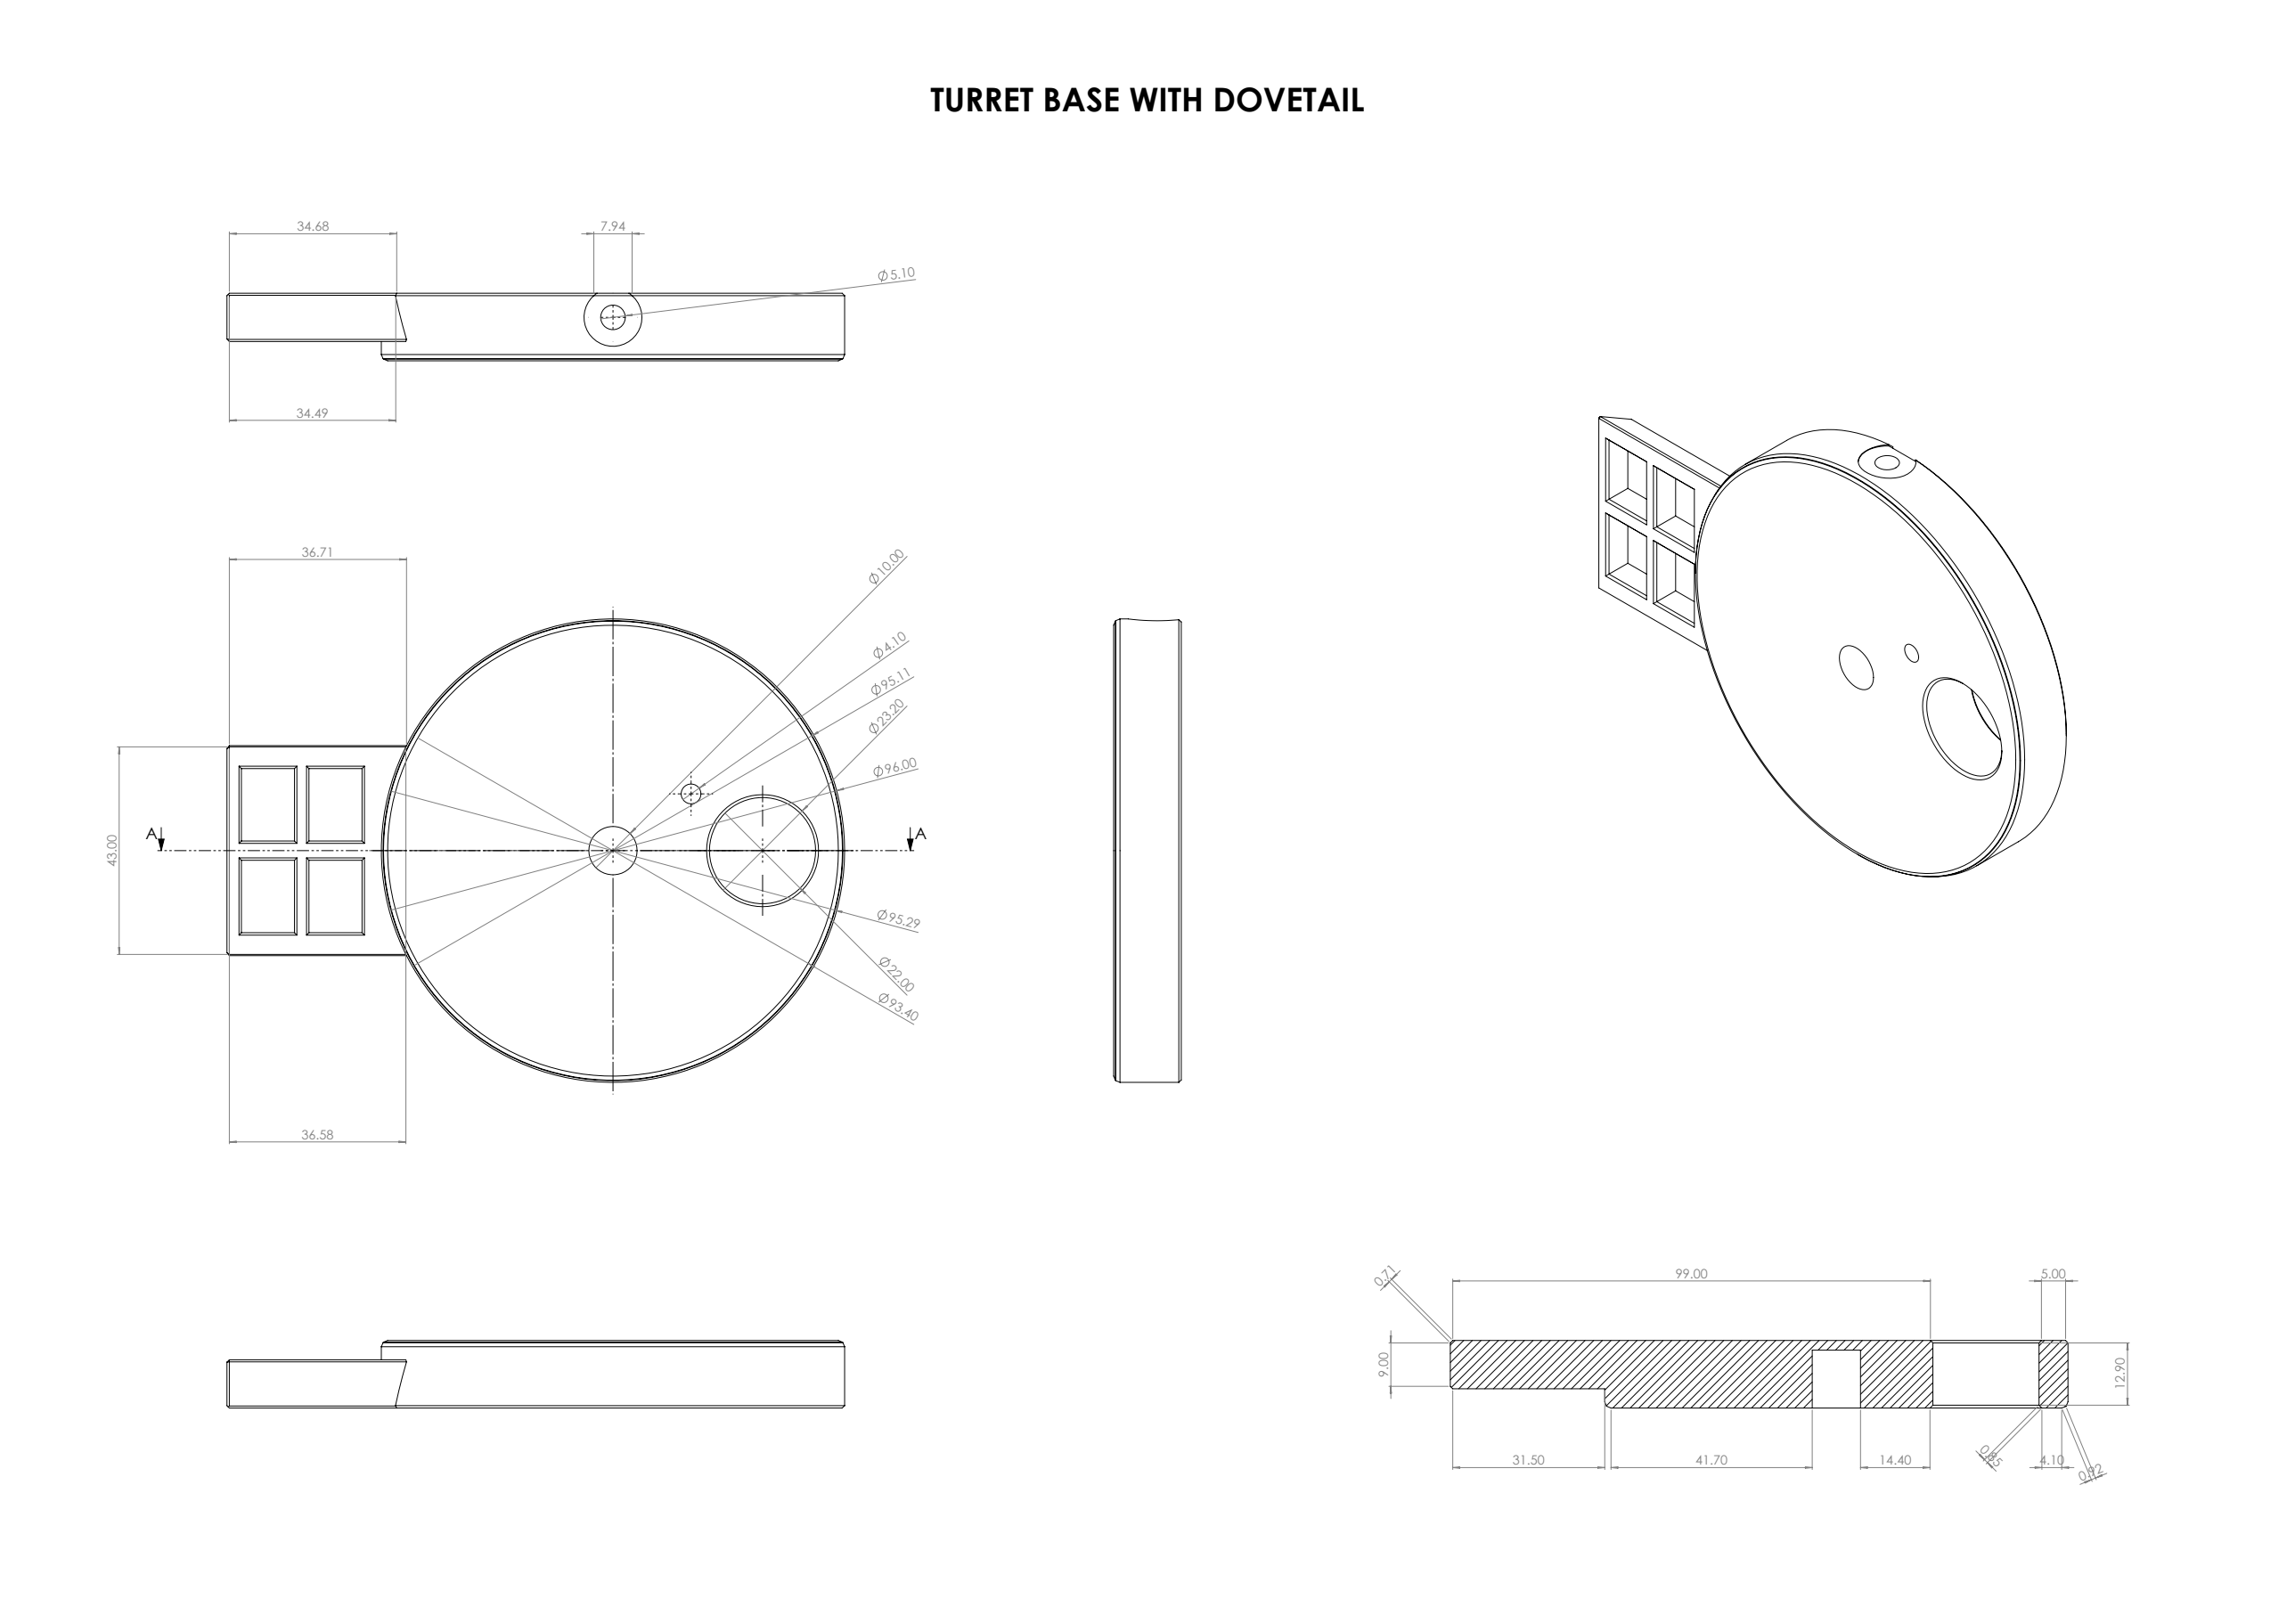
ISO-10303-21;
HEADER;
/* Generated by software containing ST-Developer
 * from STEP Tools, Inc. (www.steptools.com) 
 */

FILE_DESCRIPTION(
/* description */ (''),
/* implementation_level */ '2;1');

FILE_NAME(
/* name */ '01_Turret_Base_with_Dovetail.step',
/* time_stamp */ '2026-10-21T02:03:06-07:00',
/* author */ (''),
/* organization */ (''),
/* preprocessor_version */ 'ST-DEVELOPER v20.2',
/* originating_system */ 'Autodesk Translation Framework v15.15.0.0',
/* authorisation */ '');

FILE_SCHEMA (('AUTOMOTIVE_DESIGN { 1 0 10303 214 3 1 1 }'));
ENDSEC;

DATA;
#10=MECHANICAL_DESIGN_GEOMETRIC_PRESENTATION_REPRESENTATION('',(#115),#38528);
#91=SHAPE_REPRESENTATION_RELATIONSHIP('SRR','None',#38576,#103);
#103=ADVANCED_BREP_SHAPE_REPRESENTATION('',(#127),#38516);
#115=STYLED_ITEM('',(#38685),#127);
#127=MANIFOLD_SOLID_BREP('Body1',#17072);
#139=CYLINDRICAL_SURFACE('',#17258,6.);
#140=CYLINDRICAL_SURFACE('',#17281,2.55);
#141=CYLINDRICAL_SURFACE('',#17296,48.);
#142=CYLINDRICAL_SURFACE('',#17299,11.);
#143=CYLINDRICAL_SURFACE('',#17308,2.55);
#144=CYLINDRICAL_SURFACE('',#17313,2.05);
#145=CYLINDRICAL_SURFACE('',#17314,5.);
#428=B_SPLINE_CURVE_WITH_KNOTS('',3,(#23818,#23819,#23820,#23821,#23822,
#23823),.UNSPECIFIED.,.F.,.F.,(4,2,4),(2.30648016522772,2.36442361206073,
2.39897284114794),.UNSPECIFIED.);
#429=B_SPLINE_CURVE_WITH_KNOTS('',3,(#23838,#23839,#23840,#23841,#23842,
#23843),.UNSPECIFIED.,.F.,.F.,(4,2,4),(1.51323695998699,1.54778618907421,
1.60572963590723),.UNSPECIFIED.);
#430=B_SPLINE_CURVE_WITH_KNOTS('',3,(#23844,#23845,#23846,#23847,#23848,
#23849,#23850,#23851,#23852,#23853,#23854,#23855,#23856,#23857,#23858,#23859,
#23860,#23861,#23862,#23863,#23864,#23865,#23866,#23867,#23868,#23869,#23870,
#23871,#23872,#23873,#23874),.UNSPECIFIED.,.F.,.F.,(4,2,2,3,2,2,2,2,2,2,
2,2,2,2,4),(-0.489813721019733,-0.452534469426352,-0.226267234713176,0.,
0.226267234713176,0.452534469426352,0.678799813883625,0.905065158340898,
1.13133050279817,1.35759584725544,1.58386308196862,1.8101303166818,2.03639755139497,
2.26266478610815,2.29994403770815),.UNSPECIFIED.);
#847=CONICAL_SURFACE('',#17255,47.75,0.785398163397447);
#848=CONICAL_SURFACE('',#17266,47.75,0.785398163397447);
#849=CONICAL_SURFACE('',#17279,2.8,0.785398163397449);
#850=CONICAL_SURFACE('',#17291,47.8232233047034,0.392699081698724);
#851=CONICAL_SURFACE('',#17294,47.6,0.785398163397448);
#852=CONICAL_SURFACE('',#17297,11.25,0.785398163397446);
#853=CONICAL_SURFACE('',#17301,47.1267766952966,1.17809724509617);
#854=CONICAL_SURFACE('',#17307,11.3,0.785398163397444);
#1051=(
BOUNDED_CURVE()
B_SPLINE_CURVE(2,(#23805,#23806,#23807),.UNSPECIFIED.,.F.,.F.)
B_SPLINE_CURVE_WITH_KNOTS((3,3),(0.207879657438984,0.217458646013456),
 .UNSPECIFIED.)
CURVE()
GEOMETRIC_REPRESENTATION_ITEM()
RATIONAL_B_SPLINE_CURVE((1.00012625079627,1.0001251588785,1.00012369825994))
REPRESENTATION_ITEM('')
);
#1052=(
BOUNDED_CURVE()
B_SPLINE_CURVE(2,(#23889,#23890,#23891),.UNSPECIFIED.,.F.,.F.)
B_SPLINE_CURVE_WITH_KNOTS((3,3),(0.141563780335619,0.151142768910042),
 .UNSPECIFIED.)
CURVE()
GEOMETRIC_REPRESENTATION_ITEM()
RATIONAL_B_SPLINE_CURVE((1.00012369825443,1.00012515887293,1.00012625079065))
REPRESENTATION_ITEM('')
);
#1424=ELLIPSE('',#17244,96.0000000000002,48.);
#1425=ELLIPSE('',#17247,96.0000000000002,48.);
#1426=ELLIPSE('',#17252,96.,48.);
#1427=ELLIPSE('',#17254,66.5459160514177,47.0550685002283);
#1428=ELLIPSE('',#17259,8.48528137423855,6.);
#1429=ELLIPSE('',#17261,8.48528137423855,6.);
#1430=ELLIPSE('',#17268,66.5459160514174,47.0550685002282);
#1431=ELLIPSE('',#17285,96.,48.);
#1432=FACE_BOUND('',#3270,.T.);
#1433=FACE_BOUND('',#3271,.T.);
#1434=FACE_BOUND('',#3272,.T.);
#1435=FACE_BOUND('',#3273,.T.);
#1436=FACE_BOUND('',#3300,.T.);
#1437=FACE_BOUND('',#3301,.T.);
#1438=FACE_BOUND('',#3321,.T.);
#1439=FACE_BOUND('',#3329,.T.);
#1440=FACE_BOUND('',#3330,.T.);
#1441=FACE_BOUND('',#3331,.T.);
#1442=FACE_BOUND('',#3336,.T.);
#1477=CIRCLE('',#17226,48.);
#1478=CIRCLE('',#17227,48.);
#1479=CIRCLE('',#17256,48.);
#1480=CIRCLE('',#17257,47.5);
#1481=CIRCLE('',#17260,6.);
#1482=CIRCLE('',#17263,47.5);
#1483=CIRCLE('',#17264,3.05);
#1484=CIRCLE('',#17265,11.5);
#1485=CIRCLE('',#17267,48.);
#1486=CIRCLE('',#17280,2.55);
#1487=CIRCLE('',#17282,2.55);
#1488=CIRCLE('',#17290,2.55);
#1489=CIRCLE('',#17292,47.6464466094067);
#1490=CIRCLE('',#17293,48.);
#1491=CIRCLE('',#17295,47.5535533905933);
#1492=CIRCLE('',#17298,11.);
#1493=CIRCLE('',#17300,11.);
#1494=CIRCLE('',#17302,46.7);
#1495=CIRCLE('',#17304,11.6);
#1496=CIRCLE('',#17305,5.);
#1497=CIRCLE('',#17306,2.05);
#1498=CIRCLE('',#17309,2.55);
#1499=CIRCLE('',#17312,2.05);
#1500=CIRCLE('',#17315,5.);
#2280=FACE_OUTER_BOUND('',#3263,.T.);
#2281=FACE_OUTER_BOUND('',#3264,.T.);
#2282=FACE_OUTER_BOUND('',#3265,.T.);
#2283=FACE_OUTER_BOUND('',#3266,.T.);
#2284=FACE_OUTER_BOUND('',#3267,.T.);
#2285=FACE_OUTER_BOUND('',#3268,.T.);
#2286=FACE_OUTER_BOUND('',#3269,.T.);
#2287=FACE_OUTER_BOUND('',#3274,.T.);
#2288=FACE_OUTER_BOUND('',#3275,.T.);
#2289=FACE_OUTER_BOUND('',#3276,.T.);
#2290=FACE_OUTER_BOUND('',#3277,.T.);
#2291=FACE_OUTER_BOUND('',#3278,.T.);
#2292=FACE_OUTER_BOUND('',#3279,.T.);
#2293=FACE_OUTER_BOUND('',#3280,.T.);
#2294=FACE_OUTER_BOUND('',#3281,.T.);
#2295=FACE_OUTER_BOUND('',#3282,.T.);
#2296=FACE_OUTER_BOUND('',#3283,.T.);
#2297=FACE_OUTER_BOUND('',#3284,.T.);
#2298=FACE_OUTER_BOUND('',#3285,.T.);
#2299=FACE_OUTER_BOUND('',#3286,.T.);
#2300=FACE_OUTER_BOUND('',#3287,.T.);
#2301=FACE_OUTER_BOUND('',#3288,.T.);
#2302=FACE_OUTER_BOUND('',#3289,.T.);
#2303=FACE_OUTER_BOUND('',#3290,.T.);
#2304=FACE_OUTER_BOUND('',#3291,.T.);
#2305=FACE_OUTER_BOUND('',#3292,.T.);
#2306=FACE_OUTER_BOUND('',#3293,.T.);
#2307=FACE_OUTER_BOUND('',#3294,.T.);
#2308=FACE_OUTER_BOUND('',#3295,.T.);
#2309=FACE_OUTER_BOUND('',#3296,.T.);
#2310=FACE_OUTER_BOUND('',#3297,.T.);
#2311=FACE_OUTER_BOUND('',#3298,.T.);
#2312=FACE_OUTER_BOUND('',#3299,.T.);
#2313=FACE_OUTER_BOUND('',#3302,.T.);
#2314=FACE_OUTER_BOUND('',#3303,.T.);
#2315=FACE_OUTER_BOUND('',#3304,.T.);
#2316=FACE_OUTER_BOUND('',#3305,.T.);
#2317=FACE_OUTER_BOUND('',#3306,.T.);
#2318=FACE_OUTER_BOUND('',#3307,.T.);
#2319=FACE_OUTER_BOUND('',#3308,.T.);
#2320=FACE_OUTER_BOUND('',#3309,.T.);
#2321=FACE_OUTER_BOUND('',#3310,.T.);
#2322=FACE_OUTER_BOUND('',#3311,.T.);
#2323=FACE_OUTER_BOUND('',#3312,.T.);
#2324=FACE_OUTER_BOUND('',#3313,.T.);
#2325=FACE_OUTER_BOUND('',#3314,.T.);
#2326=FACE_OUTER_BOUND('',#3315,.T.);
#2327=FACE_OUTER_BOUND('',#3316,.T.);
#2328=FACE_OUTER_BOUND('',#3317,.T.);
#2329=FACE_OUTER_BOUND('',#3318,.T.);
#2330=FACE_OUTER_BOUND('',#3319,.T.);
#2331=FACE_OUTER_BOUND('',#3320,.T.);
#2332=FACE_OUTER_BOUND('',#3322,.T.);
#2333=FACE_OUTER_BOUND('',#3323,.T.);
#2334=FACE_OUTER_BOUND('',#3324,.T.);
#2335=FACE_OUTER_BOUND('',#3325,.T.);
#2336=FACE_OUTER_BOUND('',#3326,.T.);
#2337=FACE_OUTER_BOUND('',#3327,.T.);
#2338=FACE_OUTER_BOUND('',#3328,.T.);
#2339=FACE_OUTER_BOUND('',#3332,.T.);
#2340=FACE_OUTER_BOUND('',#3333,.T.);
#2341=FACE_OUTER_BOUND('',#3334,.T.);
#2342=FACE_OUTER_BOUND('',#3335,.T.);
#2343=FACE_OUTER_BOUND('',#3337,.T.);
#2344=FACE_OUTER_BOUND('',#3338,.T.);
#2345=FACE_OUTER_BOUND('',#3339,.T.);
#2346=FACE_OUTER_BOUND('',#3340,.T.);
#2347=FACE_OUTER_BOUND('',#3341,.T.);
#2348=FACE_OUTER_BOUND('',#3342,.T.);
#2349=FACE_OUTER_BOUND('',#3343,.T.);
#2350=FACE_OUTER_BOUND('',#3344,.T.);
#2351=FACE_OUTER_BOUND('',#3345,.T.);
#3263=EDGE_LOOP('',(#10459,#10460,#10461,#10462));
#3264=EDGE_LOOP('',(#10463,#10464,#10465,#10466));
#3265=EDGE_LOOP('',(#10467,#10468,#10469,#10470));
#3266=EDGE_LOOP('',(#10471,#10472,#10473,#10474));
#3267=EDGE_LOOP('',(#10475,#10476,#10477,#10478));
#3268=EDGE_LOOP('',(#10479,#10480,#10481,#10482));
#3269=EDGE_LOOP('',(#10483,#10484,#10485,#10486,#10487));
#3270=EDGE_LOOP('',(#10488,#10489,#10490,#10491));
#3271=EDGE_LOOP('',(#10492,#10493,#10494,#10495));
#3272=EDGE_LOOP('',(#10496,#10497,#10498,#10499));
#3273=EDGE_LOOP('',(#10500,#10501,#10502,#10503));
#3274=EDGE_LOOP('',(#10504,#10505,#10506,#10507));
#3275=EDGE_LOOP('',(#10508,#10509,#10510,#10511));
#3276=EDGE_LOOP('',(#10512,#10513,#10514,#10515));
#3277=EDGE_LOOP('',(#10516,#10517,#10518,#10519));
#3278=EDGE_LOOP('',(#10520,#10521,#10522,#10523));
#3279=EDGE_LOOP('',(#10524,#10525,#10526,#10527));
#3280=EDGE_LOOP('',(#10528,#10529,#10530,#10531));
#3281=EDGE_LOOP('',(#10532,#10533,#10534,#10535));
#3282=EDGE_LOOP('',(#10536,#10537,#10538,#10539));
#3283=EDGE_LOOP('',(#10540,#10541,#10542,#10543));
#3284=EDGE_LOOP('',(#10544,#10545,#10546,#10547));
#3285=EDGE_LOOP('',(#10548,#10549,#10550,#10551));
#3286=EDGE_LOOP('',(#10552,#10553,#10554,#10555));
#3287=EDGE_LOOP('',(#10556,#10557,#10558,#10559));
#3288=EDGE_LOOP('',(#10560,#10561,#10562));
#3289=EDGE_LOOP('',(#10563,#10564,#10565,#10566));
#3290=EDGE_LOOP('',(#10567,#10568,#10569));
#3291=EDGE_LOOP('',(#10570,#10571,#10572,#10573));
#3292=EDGE_LOOP('',(#10574,#10575,#10576,#10577,#10578));
#3293=EDGE_LOOP('',(#10579,#10580,#10581,#10582));
#3294=EDGE_LOOP('',(#10583,#10584,#10585,#10586,#10587));
#3295=EDGE_LOOP('',(#10588,#10589,#10590,#10591,#10592));
#3296=EDGE_LOOP('',(#10593,#10594,#10595,#10596,#10597));
#3297=EDGE_LOOP('',(#10598,#10599,#10600,#10601,#10602));
#3298=EDGE_LOOP('',(#10603,#10604,#10605,#10606,#10607,#10608,#10609,#10610));
#3299=EDGE_LOOP('',(#10611,#10612,#10613,#10614,#10615,#10616,#10617,#10618));
#3300=EDGE_LOOP('',(#10619));
#3301=EDGE_LOOP('',(#10620));
#3302=EDGE_LOOP('',(#10621,#10622,#10623,#10624,#10625));
#3303=EDGE_LOOP('',(#10626,#10627,#10628,#10629));
#3304=EDGE_LOOP('',(#10630,#10631,#10632,#10633));
#3305=EDGE_LOOP('',(#10634,#10635,#10636,#10637));
#3306=EDGE_LOOP('',(#10638,#10639,#10640,#10641));
#3307=EDGE_LOOP('',(#10642,#10643,#10644,#10645));
#3308=EDGE_LOOP('',(#10646,#10647,#10648,#10649));
#3309=EDGE_LOOP('',(#10650,#10651,#10652,#10653));
#3310=EDGE_LOOP('',(#10654,#10655,#10656,#10657));
#3311=EDGE_LOOP('',(#10658,#10659,#10660,#10661));
#3312=EDGE_LOOP('',(#10662,#10663,#10664,#10665));
#3313=EDGE_LOOP('',(#10666,#10667,#10668,#10669));
#3314=EDGE_LOOP('',(#10670,#10671,#10672,#10673));
#3315=EDGE_LOOP('',(#10674,#10675,#10676,#10677,#10678));
#3316=EDGE_LOOP('',(#10679,#10680,#10681,#10682,#10683));
#3317=EDGE_LOOP('',(#10684,#10685,#10686,#10687,#10688,#10689));
#3318=EDGE_LOOP('',(#10690,#10691,#10692,#10693));
#3319=EDGE_LOOP('',(#10694,#10695,#10696,#10697));
#3320=EDGE_LOOP('',(#10698,#10699));
#3321=EDGE_LOOP('',(#10700));
#3322=EDGE_LOOP('',(#10701,#10702,#10703,#10704));
#3323=EDGE_LOOP('',(#10705,#10706,#10707,#10708));
#3324=EDGE_LOOP('',(#10709,#10710,#10711,#10712,#10713,#10714,#10715,#10716,
#10717,#10718,#10719,#10720));
#3325=EDGE_LOOP('',(#10721,#10722,#10723,#10724));
#3326=EDGE_LOOP('',(#10725,#10726,#10727,#10728));
#3327=EDGE_LOOP('',(#10729,#10730,#10731,#10732));
#3328=EDGE_LOOP('',(#10733));
#3329=EDGE_LOOP('',(#10734));
#3330=EDGE_LOOP('',(#10735));
#3331=EDGE_LOOP('',(#10736));
#3332=EDGE_LOOP('',(#10737,#10738,#10739,#10740));
#3333=EDGE_LOOP('',(#10741,#10742,#10743,#10744));
#3334=EDGE_LOOP('',(#10745));
#3335=EDGE_LOOP('',(#10746));
#3336=EDGE_LOOP('',(#10747));
#3337=EDGE_LOOP('',(#10748,#10749,#10750,#10751));
#3338=EDGE_LOOP('',(#10752,#10753,#10754,#10755));
#3339=EDGE_LOOP('',(#10756));
#3340=EDGE_LOOP('',(#10757,#10758,#10759,#10760));
#3341=EDGE_LOOP('',(#10761,#10762,#10763,#10764));
#3342=EDGE_LOOP('',(#10765,#10766,#10767,#10768));
#3343=EDGE_LOOP('',(#10769,#10770,#10771,#10772));
#3344=EDGE_LOOP('',(#10773,#10774,#10775,#10776));
#3345=EDGE_LOOP('',(#10777,#10778,#10779,#10780));
#4291=LINE('',#23621,#5266);
#4292=LINE('',#23623,#5267);
#4293=LINE('',#23625,#5268);
#4294=LINE('',#23626,#5269);
#4295=LINE('',#23630,#5270);
#4296=LINE('',#23632,#5271);
#4297=LINE('',#23634,#5272);
#4298=LINE('',#23635,#5273);
#4299=LINE('',#23637,#5274);
#4300=LINE('',#23638,#5275);
#4301=LINE('',#23640,#5276);
#4302=LINE('',#23641,#5277);
#4303=LINE('',#23644,#5278);
#4304=LINE('',#23646,#5279);
#4305=LINE('',#23647,#5280);
#4306=LINE('',#23650,#5281);
#4307=LINE('',#23651,#5282);
#4308=LINE('',#23655,#5283);
#4309=LINE('',#23657,#5284);
#4310=LINE('',#23659,#5285);
#4311=LINE('',#23665,#5286);
#4312=LINE('',#23667,#5287);
#4313=LINE('',#23669,#5288);
#4314=LINE('',#23670,#5289);
#4315=LINE('',#23673,#5290);
#4316=LINE('',#23675,#5291);
#4317=LINE('',#23677,#5292);
#4318=LINE('',#23678,#5293);
#4319=LINE('',#23681,#5294);
#4320=LINE('',#23683,#5295);
#4321=LINE('',#23685,#5296);
#4322=LINE('',#23686,#5297);
#4323=LINE('',#23690,#5298);
#4324=LINE('',#23691,#5299);
#4325=LINE('',#23692,#5300);
#4326=LINE('',#23695,#5301);
#4327=LINE('',#23696,#5302);
#4328=LINE('',#23699,#5303);
#4329=LINE('',#23700,#5304);
#4330=LINE('',#23703,#5305);
#4331=LINE('',#23705,#5306);
#4332=LINE('',#23706,#5307);
#4333=LINE('',#23709,#5308);
#4334=LINE('',#23710,#5309);
#4335=LINE('',#23713,#5310);
#4336=LINE('',#23714,#5311);
#4337=LINE('',#23717,#5312);
#4338=LINE('',#23719,#5313);
#4339=LINE('',#23720,#5314);
#4340=LINE('',#23723,#5315);
#4341=LINE('',#23725,#5316);
#4342=LINE('',#23726,#5317);
#4343=LINE('',#23729,#5318);
#4344=LINE('',#23731,#5319);
#4345=LINE('',#23732,#5320);
#4346=LINE('',#23735,#5321);
#4347=LINE('',#23737,#5322);
#4348=LINE('',#23738,#5323);
#4349=LINE('',#23741,#5324);
#4350=LINE('',#23743,#5325);
#4351=LINE('',#23744,#5326);
#4352=LINE('',#23747,#5327);
#4353=LINE('',#23749,#5328);
#4354=LINE('',#23750,#5329);
#4355=LINE('',#23753,#5330);
#4356=LINE('',#23755,#5331);
#4357=LINE('',#23756,#5332);
#4358=LINE('',#23759,#5333);
#4359=LINE('',#23761,#5334);
#4360=LINE('',#23762,#5335);
#4361=LINE('',#23766,#5336);
#4362=LINE('',#23767,#5337);
#4363=LINE('',#23768,#5338);
#4364=LINE('',#23772,#5339);
#4365=LINE('',#23775,#5340);
#4366=LINE('',#23777,#5341);
#4367=LINE('',#23778,#5342);
#4368=LINE('',#23782,#5343);
#4369=LINE('',#23786,#5344);
#4370=LINE('',#23787,#5345);
#4371=LINE('',#23789,#5346);
#4372=LINE('',#23790,#5347);
#4373=LINE('',#23792,#5348);
#4374=LINE('',#23796,#5349);
#4375=LINE('',#23797,#5350);
#4376=LINE('',#23799,#5351);
#4377=LINE('',#23800,#5352);
#4378=LINE('',#23803,#5353);
#4379=LINE('',#23811,#5354);
#4380=LINE('',#23813,#5355);
#4381=LINE('',#23828,#5356);
#4382=LINE('',#23836,#5357);
#4383=LINE('',#23877,#5358);
#4384=LINE('',#23879,#5359);
#4385=LINE('',#23881,#5360);
#4386=LINE('',#23895,#5361);
#4387=LINE('',#23897,#5362);
#4388=LINE('',#23899,#5363);
#4389=LINE('',#23901,#5364);
#4390=LINE('',#23903,#5365);
#4391=LINE('',#23905,#5366);
#4392=LINE('',#23907,#5367);
#4393=LINE('',#23909,#5368);
#4394=LINE('',#23911,#5369);
#4395=LINE('',#23913,#5370);
#4396=LINE('',#23916,#5371);
#4397=LINE('',#23920,#5372);
#4398=LINE('',#23923,#5373);
#4399=LINE('',#23924,#5374);
#4400=LINE('',#23928,#5375);
#4401=LINE('',#23931,#5376);
#4402=LINE('',#23939,#5377);
#4403=LINE('',#23944,#5378);
#4404=LINE('',#23946,#5379);
#4405=LINE('',#23949,#5380);
#4406=LINE('',#23954,#5381);
#4407=LINE('',#23957,#5382);
#4408=LINE('',#23967,#5383);
#4409=LINE('',#23970,#5384);
#4410=LINE('',#23977,#5385);
#4411=LINE('',#23980,#5386);
#4412=LINE('',#23988,#5387);
#4413=LINE('',#23989,#5388);
#4414=LINE('',#23991,#5389);
#5266=VECTOR('',#19031,10.);
#5267=VECTOR('',#19032,10.);
#5268=VECTOR('',#19033,10.);
#5269=VECTOR('',#19034,10.);
#5270=VECTOR('',#19037,10.);
#5271=VECTOR('',#19038,10.);
#5272=VECTOR('',#19039,10.);
#5273=VECTOR('',#19040,10.);
#5274=VECTOR('',#19043,10.);
#5275=VECTOR('',#19044,10.);
#5276=VECTOR('',#19047,10.);
#5277=VECTOR('',#19048,10.);
#5278=VECTOR('',#19051,10.);
#5279=VECTOR('',#19052,10.);
#5280=VECTOR('',#19053,10.);
#5281=VECTOR('',#19056,10.);
#5282=VECTOR('',#19057,10.);
#5283=VECTOR('',#19060,10.);
#5284=VECTOR('',#19061,10.);
#5285=VECTOR('',#19062,10.);
#5286=VECTOR('',#19067,10.);
#5287=VECTOR('',#19068,10.);
#5288=VECTOR('',#19069,10.);
#5289=VECTOR('',#19070,10.);
#5290=VECTOR('',#19071,10.);
#5291=VECTOR('',#19072,10.);
#5292=VECTOR('',#19073,10.);
#5293=VECTOR('',#19074,10.);
#5294=VECTOR('',#19075,10.);
#5295=VECTOR('',#19076,10.);
#5296=VECTOR('',#19077,10.);
#5297=VECTOR('',#19078,10.);
#5298=VECTOR('',#19081,10.);
#5299=VECTOR('',#19082,10.);
#5300=VECTOR('',#19083,10.);
#5301=VECTOR('',#19086,10.);
#5302=VECTOR('',#19087,10.);
#5303=VECTOR('',#19090,10.);
#5304=VECTOR('',#19091,10.);
#5305=VECTOR('',#19094,10.);
#5306=VECTOR('',#19095,10.);
#5307=VECTOR('',#19096,10.);
#5308=VECTOR('',#19099,10.);
#5309=VECTOR('',#19100,10.);
#5310=VECTOR('',#19103,10.);
#5311=VECTOR('',#19104,10.);
#5312=VECTOR('',#19107,10.);
#5313=VECTOR('',#19108,10.);
#5314=VECTOR('',#19109,10.);
#5315=VECTOR('',#19112,10.);
#5316=VECTOR('',#19113,10.);
#5317=VECTOR('',#19114,10.);
#5318=VECTOR('',#19117,10.);
#5319=VECTOR('',#19118,10.);
#5320=VECTOR('',#19119,10.);
#5321=VECTOR('',#19122,10.);
#5322=VECTOR('',#19123,10.);
#5323=VECTOR('',#19124,10.);
#5324=VECTOR('',#19127,10.);
#5325=VECTOR('',#19128,10.);
#5326=VECTOR('',#19129,10.);
#5327=VECTOR('',#19132,10.);
#5328=VECTOR('',#19133,10.);
#5329=VECTOR('',#19134,10.);
#5330=VECTOR('',#19137,10.);
#5331=VECTOR('',#19138,10.);
#5332=VECTOR('',#19139,10.);
#5333=VECTOR('',#19142,10.);
#5334=VECTOR('',#19143,10.);
#5335=VECTOR('',#19144,10.);
#5336=VECTOR('',#19147,10.);
#5337=VECTOR('',#19148,10.);
#5338=VECTOR('',#19149,10.);
#5339=VECTOR('',#19154,10.);
#5340=VECTOR('',#19157,10.);
#5341=VECTOR('',#19158,10.);
#5342=VECTOR('',#19159,10.);
#5343=VECTOR('',#19164,10.);
#5344=VECTOR('',#19167,10.);
#5345=VECTOR('',#19168,10.);
#5346=VECTOR('',#19169,10.);
#5347=VECTOR('',#19170,10.);
#5348=VECTOR('',#19173,10.);
#5349=VECTOR('',#19176,10.);
#5350=VECTOR('',#19177,10.);
#5351=VECTOR('',#19178,10.);
#5352=VECTOR('',#19179,10.);
#5353=VECTOR('',#19182,10.);
#5354=VECTOR('',#19187,10.);
#5355=VECTOR('',#19188,10.);
#5356=VECTOR('',#19199,10.);
#5357=VECTOR('',#19206,10.);
#5358=VECTOR('',#19209,10.);
#5359=VECTOR('',#19210,10.);
#5360=VECTOR('',#19213,10.);
#5361=VECTOR('',#19226,10.);
#5362=VECTOR('',#19229,10.);
#5363=VECTOR('',#19232,10.);
#5364=VECTOR('',#19235,10.);
#5365=VECTOR('',#19238,10.);
#5366=VECTOR('',#19241,10.);
#5367=VECTOR('',#19244,10.);
#5368=VECTOR('',#19247,10.);
#5369=VECTOR('',#19250,10.);
#5370=VECTOR('',#19253,10.);
#5371=VECTOR('',#19256,2.8);
#5372=VECTOR('',#19261,2.55);
#5373=VECTOR('',#19266,10.);
#5374=VECTOR('',#19267,10.);
#5375=VECTOR('',#19274,10.);
#5376=VECTOR('',#19279,10.);
#5377=VECTOR('',#19288,47.8232233047034);
#5378=VECTOR('',#19295,47.6);
#5379=VECTOR('',#19298,48.);
#5380=VECTOR('',#19301,11.25);
#5381=VECTOR('',#19308,11.);
#5382=VECTOR('',#19311,47.1267766952966);
#5383=VECTOR('',#19324,11.3);
#5384=VECTOR('',#19327,2.55);
#5385=VECTOR('',#19338,2.05);
#5386=VECTOR('',#19341,5.);
#5387=VECTOR('',#19354,10.);
#5388=VECTOR('',#19355,10.);
#5389=VECTOR('',#19358,10.);
#6241=VERTEX_POINT('',#23619);
#6242=VERTEX_POINT('',#23620);
#6243=VERTEX_POINT('',#23622);
#6244=VERTEX_POINT('',#23624);
#6245=VERTEX_POINT('',#23628);
#6246=VERTEX_POINT('',#23629);
#6247=VERTEX_POINT('',#23631);
#6248=VERTEX_POINT('',#23633);
#6249=VERTEX_POINT('',#23643);
#6250=VERTEX_POINT('',#23645);
#6251=VERTEX_POINT('',#23649);
#6252=VERTEX_POINT('',#23653);
#6253=VERTEX_POINT('',#23654);
#6254=VERTEX_POINT('',#23656);
#6255=VERTEX_POINT('',#23658);
#6256=VERTEX_POINT('',#23660);
#6257=VERTEX_POINT('',#23663);
#6258=VERTEX_POINT('',#23664);
#6259=VERTEX_POINT('',#23666);
#6260=VERTEX_POINT('',#23668);
#6261=VERTEX_POINT('',#23671);
#6262=VERTEX_POINT('',#23672);
#6263=VERTEX_POINT('',#23674);
#6264=VERTEX_POINT('',#23676);
#6265=VERTEX_POINT('',#23679);
#6266=VERTEX_POINT('',#23680);
#6267=VERTEX_POINT('',#23682);
#6268=VERTEX_POINT('',#23684);
#6269=VERTEX_POINT('',#23688);
#6270=VERTEX_POINT('',#23689);
#6271=VERTEX_POINT('',#23694);
#6272=VERTEX_POINT('',#23698);
#6273=VERTEX_POINT('',#23702);
#6274=VERTEX_POINT('',#23704);
#6275=VERTEX_POINT('',#23708);
#6276=VERTEX_POINT('',#23712);
#6277=VERTEX_POINT('',#23716);
#6278=VERTEX_POINT('',#23718);
#6279=VERTEX_POINT('',#23722);
#6280=VERTEX_POINT('',#23724);
#6281=VERTEX_POINT('',#23728);
#6282=VERTEX_POINT('',#23730);
#6283=VERTEX_POINT('',#23734);
#6284=VERTEX_POINT('',#23736);
#6285=VERTEX_POINT('',#23740);
#6286=VERTEX_POINT('',#23742);
#6287=VERTEX_POINT('',#23746);
#6288=VERTEX_POINT('',#23748);
#6289=VERTEX_POINT('',#23752);
#6290=VERTEX_POINT('',#23754);
#6291=VERTEX_POINT('',#23758);
#6292=VERTEX_POINT('',#23760);
#6293=VERTEX_POINT('',#23764);
#6294=VERTEX_POINT('',#23765);
#6295=VERTEX_POINT('',#23770);
#6296=VERTEX_POINT('',#23774);
#6297=VERTEX_POINT('',#23776);
#6298=VERTEX_POINT('',#23780);
#6299=VERTEX_POINT('',#23784);
#6300=VERTEX_POINT('',#23785);
#6301=VERTEX_POINT('',#23788);
#6302=VERTEX_POINT('',#23794);
#6303=VERTEX_POINT('',#23795);
#6304=VERTEX_POINT('',#23798);
#6305=VERTEX_POINT('',#23802);
#6306=VERTEX_POINT('',#23804);
#6307=VERTEX_POINT('',#23810);
#6308=VERTEX_POINT('',#23812);
#6309=VERTEX_POINT('',#23816);
#6310=VERTEX_POINT('',#23817);
#6311=VERTEX_POINT('',#23827);
#6312=VERTEX_POINT('',#23829);
#6313=VERTEX_POINT('',#23831);
#6314=VERTEX_POINT('',#23833);
#6315=VERTEX_POINT('',#23835);
#6316=VERTEX_POINT('',#23837);
#6317=VERTEX_POINT('',#23876);
#6318=VERTEX_POINT('',#23878);
#6319=VERTEX_POINT('',#23882);
#6320=VERTEX_POINT('',#23884);
#6321=VERTEX_POINT('',#23887);
#6322=VERTEX_POINT('',#23888);
#6323=VERTEX_POINT('',#23915);
#6324=VERTEX_POINT('',#23919);
#6325=VERTEX_POINT('',#23933);
#6326=VERTEX_POINT('',#23936);
#6327=VERTEX_POINT('',#23938);
#6328=VERTEX_POINT('',#23942);
#6329=VERTEX_POINT('',#23948);
#6330=VERTEX_POINT('',#23952);
#6331=VERTEX_POINT('',#23956);
#6332=VERTEX_POINT('',#23960);
#6333=VERTEX_POINT('',#23962);
#6334=VERTEX_POINT('',#23964);
#6335=VERTEX_POINT('',#23969);
#6336=VERTEX_POINT('',#23974);
#6337=VERTEX_POINT('',#23979);
#6338=VERTEX_POINT('',#23987);
#7881=EDGE_CURVE('',#6241,#6242,#4291,.T.);
#7882=EDGE_CURVE('',#6242,#6243,#4292,.T.);
#7883=EDGE_CURVE('',#6243,#6244,#4293,.T.);
#7884=EDGE_CURVE('',#6241,#6244,#4294,.T.);
#7885=EDGE_CURVE('',#6245,#6246,#4295,.T.);
#7886=EDGE_CURVE('',#6246,#6247,#4296,.T.);
#7887=EDGE_CURVE('',#6247,#6248,#4297,.T.);
#7888=EDGE_CURVE('',#6248,#6245,#4298,.T.);
#7889=EDGE_CURVE('',#6244,#6247,#4299,.T.);
#7890=EDGE_CURVE('',#6246,#6241,#4300,.T.);
#7891=EDGE_CURVE('',#6242,#6245,#4301,.T.);
#7892=EDGE_CURVE('',#6248,#6243,#4302,.T.);
#7893=EDGE_CURVE('',#6248,#6249,#4303,.T.);
#7894=EDGE_CURVE('',#6249,#6250,#4304,.T.);
#7895=EDGE_CURVE('',#6243,#6250,#4305,.T.);
#7896=EDGE_CURVE('',#6247,#6251,#4306,.T.);
#7897=EDGE_CURVE('',#6251,#6249,#4307,.T.);
#7898=EDGE_CURVE('',#6252,#6253,#4308,.T.);
#7899=EDGE_CURVE('',#6254,#6252,#4309,.T.);
#7900=EDGE_CURVE('',#6255,#6254,#4310,.T.);
#7901=EDGE_CURVE('',#6256,#6255,#1477,.T.);
#7902=EDGE_CURVE('',#6253,#6256,#1478,.T.);
#7903=EDGE_CURVE('',#6257,#6258,#4311,.T.);
#7904=EDGE_CURVE('',#6259,#6257,#4312,.T.);
#7905=EDGE_CURVE('',#6260,#6259,#4313,.T.);
#7906=EDGE_CURVE('',#6258,#6260,#4314,.T.);
#7907=EDGE_CURVE('',#6261,#6262,#4315,.T.);
#7908=EDGE_CURVE('',#6263,#6261,#4316,.T.);
#7909=EDGE_CURVE('',#6264,#6263,#4317,.T.);
#7910=EDGE_CURVE('',#6262,#6264,#4318,.T.);
#7911=EDGE_CURVE('',#6265,#6266,#4319,.T.);
#7912=EDGE_CURVE('',#6267,#6265,#4320,.T.);
#7913=EDGE_CURVE('',#6268,#6267,#4321,.T.);
#7914=EDGE_CURVE('',#6266,#6268,#4322,.T.);
#7915=EDGE_CURVE('',#6269,#6270,#4323,.T.);
#7916=EDGE_CURVE('',#6270,#6266,#4324,.F.);
#7917=EDGE_CURVE('',#6268,#6269,#4325,.T.);
#7918=EDGE_CURVE('',#6271,#6269,#4326,.T.);
#7919=EDGE_CURVE('',#6267,#6271,#4327,.T.);
#7920=EDGE_CURVE('',#6265,#6272,#4328,.F.);
#7921=EDGE_CURVE('',#6272,#6271,#4329,.T.);
#7922=EDGE_CURVE('',#6269,#6273,#4330,.T.);
#7923=EDGE_CURVE('',#6273,#6274,#4331,.T.);
#7924=EDGE_CURVE('',#6270,#6274,#4332,.T.);
#7925=EDGE_CURVE('',#6271,#6275,#4333,.T.);
#7926=EDGE_CURVE('',#6275,#6273,#4334,.T.);
#7927=EDGE_CURVE('',#6272,#6276,#4335,.T.);
#7928=EDGE_CURVE('',#6276,#6275,#4336,.T.);
#7929=EDGE_CURVE('',#6264,#6277,#4337,.F.);
#7930=EDGE_CURVE('',#6277,#6278,#4338,.T.);
#7931=EDGE_CURVE('',#6278,#6262,#4339,.F.);
#7932=EDGE_CURVE('',#6277,#6279,#4340,.T.);
#7933=EDGE_CURVE('',#6279,#6280,#4341,.T.);
#7934=EDGE_CURVE('',#6278,#6280,#4342,.T.);
#7935=EDGE_CURVE('',#6261,#6281,#4343,.F.);
#7936=EDGE_CURVE('',#6281,#6282,#4344,.T.);
#7937=EDGE_CURVE('',#6282,#6263,#4345,.F.);
#7938=EDGE_CURVE('',#6281,#6283,#4346,.T.);
#7939=EDGE_CURVE('',#6283,#6284,#4347,.T.);
#7940=EDGE_CURVE('',#6282,#6284,#4348,.T.);
#7941=EDGE_CURVE('',#6260,#6285,#4349,.F.);
#7942=EDGE_CURVE('',#6285,#6286,#4350,.T.);
#7943=EDGE_CURVE('',#6286,#6258,#4351,.F.);
#7944=EDGE_CURVE('',#6285,#6287,#4352,.T.);
#7945=EDGE_CURVE('',#6287,#6288,#4353,.T.);
#7946=EDGE_CURVE('',#6286,#6288,#4354,.T.);
#7947=EDGE_CURVE('',#6257,#6289,#4355,.F.);
#7948=EDGE_CURVE('',#6289,#6290,#4356,.T.);
#7949=EDGE_CURVE('',#6290,#6259,#4357,.F.);
#7950=EDGE_CURVE('',#6289,#6291,#4358,.T.);
#7951=EDGE_CURVE('',#6291,#6292,#4359,.T.);
#7952=EDGE_CURVE('',#6290,#6292,#4360,.T.);
#7953=EDGE_CURVE('',#6293,#6294,#4361,.T.);
#7954=EDGE_CURVE('',#6254,#6293,#4362,.T.);
#7955=EDGE_CURVE('',#6294,#6254,#4363,.T.);
#7956=EDGE_CURVE('',#6295,#6255,#1424,.F.);
#7957=EDGE_CURVE('',#6293,#6295,#4364,.T.);
#7958=EDGE_CURVE('',#6252,#6296,#4365,.T.);
#7959=EDGE_CURVE('',#6297,#6252,#4366,.T.);
#7960=EDGE_CURVE('',#6296,#6297,#4367,.T.);
#7961=EDGE_CURVE('',#6253,#6298,#1425,.F.);
#7962=EDGE_CURVE('',#6298,#6297,#4368,.T.);
#7963=EDGE_CURVE('',#6299,#6300,#4369,.T.);
#7964=EDGE_CURVE('',#6300,#6296,#4370,.T.);
#7965=EDGE_CURVE('',#6297,#6301,#4371,.T.);
#7966=EDGE_CURVE('',#6301,#6299,#4372,.T.);
#7967=EDGE_CURVE('',#6296,#6294,#4373,.T.);
#7968=EDGE_CURVE('',#6302,#6303,#4374,.T.);
#7969=EDGE_CURVE('',#6303,#6293,#4375,.T.);
#7970=EDGE_CURVE('',#6294,#6304,#4376,.T.);
#7971=EDGE_CURVE('',#6304,#6302,#4377,.T.);
#7972=EDGE_CURVE('',#6305,#6303,#4378,.T.);
#7973=EDGE_CURVE('',#6305,#6306,#1051,.T.);
#7974=EDGE_CURVE('',#6295,#6306,#1426,.T.);
#7975=EDGE_CURVE('',#6307,#6302,#4379,.T.);
#7976=EDGE_CURVE('',#6307,#6308,#4380,.T.);
#7977=EDGE_CURVE('',#6308,#6305,#1427,.T.);
#7978=EDGE_CURVE('',#6309,#6310,#428,.T.);
#7979=EDGE_CURVE('',#6310,#6306,#1479,.T.);
#7980=EDGE_CURVE('',#6308,#6309,#1480,.T.);
#7981=EDGE_CURVE('',#6311,#6309,#4381,.T.);
#7982=EDGE_CURVE('',#6312,#6311,#1428,.F.);
#7983=EDGE_CURVE('',#6312,#6313,#1481,.T.);
#7984=EDGE_CURVE('',#6314,#6313,#1429,.F.);
#7985=EDGE_CURVE('',#6315,#6314,#4382,.T.);
#7986=EDGE_CURVE('',#6316,#6315,#429,.T.);
#7987=EDGE_CURVE('',#6310,#6316,#430,.T.);
#7988=EDGE_CURVE('',#6317,#6307,#4383,.T.);
#7989=EDGE_CURVE('',#6318,#6317,#4384,.T.);
#7990=EDGE_CURVE('',#6315,#6318,#1482,.T.);
#7991=EDGE_CURVE('',#6311,#6314,#4385,.T.);
#7992=EDGE_CURVE('',#6319,#6319,#1483,.T.);
#7993=EDGE_CURVE('',#6320,#6320,#1484,.T.);
#7994=EDGE_CURVE('',#6321,#6322,#1052,.F.);
#7995=EDGE_CURVE('',#6322,#6316,#1485,.T.);
#7996=EDGE_CURVE('',#6318,#6321,#1430,.F.);
#7997=EDGE_CURVE('',#6270,#6272,#4386,.T.);
#7998=EDGE_CURVE('',#6274,#6276,#4387,.T.);
#7999=EDGE_CURVE('',#6278,#6281,#4388,.T.);
#8000=EDGE_CURVE('',#6280,#6283,#4389,.T.);
#8001=EDGE_CURVE('',#6282,#6277,#4390,.T.);
#8002=EDGE_CURVE('',#6284,#6279,#4391,.T.);
#8003=EDGE_CURVE('',#6286,#6289,#4392,.T.);
#8004=EDGE_CURVE('',#6288,#6291,#4393,.T.);
#8005=EDGE_CURVE('',#6290,#6285,#4394,.T.);
#8006=EDGE_CURVE('',#6292,#6287,#4395,.T.);
#8007=EDGE_CURVE('',#6319,#6323,#4396,.T.);
#8008=EDGE_CURVE('',#6323,#6323,#1486,.T.);
#8009=EDGE_CURVE('',#6323,#6324,#4397,.T.);
#8010=EDGE_CURVE('',#6324,#6324,#1487,.T.);
#8011=EDGE_CURVE('',#6301,#6321,#4398,.T.);
#8012=EDGE_CURVE('',#6317,#6299,#4399,.T.);
#8013=EDGE_CURVE('',#6322,#6298,#1431,.T.);
#8014=EDGE_CURVE('',#6304,#6300,#4400,.T.);
#8015=EDGE_CURVE('',#6313,#6312,#4401,.T.);
#8016=EDGE_CURVE('',#6325,#6325,#1488,.T.);
#8017=EDGE_CURVE('',#6326,#6326,#1489,.T.);
#8018=EDGE_CURVE('',#6326,#6327,#4402,.T.);
#8019=EDGE_CURVE('',#6327,#6327,#1490,.T.);
#8020=EDGE_CURVE('',#6328,#6328,#1491,.T.);
#8021=EDGE_CURVE('',#6328,#6326,#4403,.T.);
#8022=EDGE_CURVE('',#6327,#6256,#4404,.T.);
#8023=EDGE_CURVE('',#6320,#6329,#4405,.T.);
#8024=EDGE_CURVE('',#6329,#6329,#1492,.T.);
#8025=EDGE_CURVE('',#6330,#6330,#1493,.T.);
#8026=EDGE_CURVE('',#6330,#6329,#4406,.T.);
#8027=EDGE_CURVE('',#6328,#6331,#4407,.T.);
#8028=EDGE_CURVE('',#6331,#6331,#1494,.T.);
#8029=EDGE_CURVE('',#6332,#6332,#1495,.T.);
#8030=EDGE_CURVE('',#6333,#6333,#1496,.T.);
#8031=EDGE_CURVE('',#6334,#6334,#1497,.T.);
#8032=EDGE_CURVE('',#6332,#6330,#4408,.T.);
#8033=EDGE_CURVE('',#6325,#6335,#4409,.T.);
#8034=EDGE_CURVE('',#6335,#6335,#1498,.T.);
#8035=EDGE_CURVE('',#6336,#6336,#1499,.T.);
#8036=EDGE_CURVE('',#6334,#6336,#4410,.T.);
#8037=EDGE_CURVE('',#6333,#6337,#4411,.T.);
#8038=EDGE_CURVE('',#6337,#6337,#1500,.T.);
#8039=EDGE_CURVE('',#6244,#6338,#4412,.T.);
#8040=EDGE_CURVE('',#6338,#6251,#4413,.T.);
#8041=EDGE_CURVE('',#6250,#6338,#4414,.T.);
#10459=ORIENTED_EDGE('',*,*,#7881,.T.);
#10460=ORIENTED_EDGE('',*,*,#7882,.T.);
#10461=ORIENTED_EDGE('',*,*,#7883,.T.);
#10462=ORIENTED_EDGE('',*,*,#7884,.F.);
#10463=ORIENTED_EDGE('',*,*,#7885,.T.);
#10464=ORIENTED_EDGE('',*,*,#7886,.T.);
#10465=ORIENTED_EDGE('',*,*,#7887,.T.);
#10466=ORIENTED_EDGE('',*,*,#7888,.T.);
#10467=ORIENTED_EDGE('',*,*,#7889,.T.);
#10468=ORIENTED_EDGE('',*,*,#7886,.F.);
#10469=ORIENTED_EDGE('',*,*,#7890,.T.);
#10470=ORIENTED_EDGE('',*,*,#7884,.T.);
#10471=ORIENTED_EDGE('',*,*,#7891,.T.);
#10472=ORIENTED_EDGE('',*,*,#7888,.F.);
#10473=ORIENTED_EDGE('',*,*,#7892,.T.);
#10474=ORIENTED_EDGE('',*,*,#7882,.F.);
#10475=ORIENTED_EDGE('',*,*,#7892,.F.);
#10476=ORIENTED_EDGE('',*,*,#7893,.T.);
#10477=ORIENTED_EDGE('',*,*,#7894,.T.);
#10478=ORIENTED_EDGE('',*,*,#7895,.F.);
#10479=ORIENTED_EDGE('',*,*,#7887,.F.);
#10480=ORIENTED_EDGE('',*,*,#7896,.T.);
#10481=ORIENTED_EDGE('',*,*,#7897,.T.);
#10482=ORIENTED_EDGE('',*,*,#7893,.F.);
#10483=ORIENTED_EDGE('',*,*,#7898,.F.);
#10484=ORIENTED_EDGE('',*,*,#7899,.F.);
#10485=ORIENTED_EDGE('',*,*,#7900,.F.);
#10486=ORIENTED_EDGE('',*,*,#7901,.F.);
#10487=ORIENTED_EDGE('',*,*,#7902,.F.);
#10488=ORIENTED_EDGE('',*,*,#7903,.F.);
#10489=ORIENTED_EDGE('',*,*,#7904,.F.);
#10490=ORIENTED_EDGE('',*,*,#7905,.F.);
#10491=ORIENTED_EDGE('',*,*,#7906,.F.);
#10492=ORIENTED_EDGE('',*,*,#7907,.F.);
#10493=ORIENTED_EDGE('',*,*,#7908,.F.);
#10494=ORIENTED_EDGE('',*,*,#7909,.F.);
#10495=ORIENTED_EDGE('',*,*,#7910,.F.);
#10496=ORIENTED_EDGE('',*,*,#7911,.F.);
#10497=ORIENTED_EDGE('',*,*,#7912,.F.);
#10498=ORIENTED_EDGE('',*,*,#7913,.F.);
#10499=ORIENTED_EDGE('',*,*,#7914,.F.);
#10500=ORIENTED_EDGE('',*,*,#7885,.F.);
#10501=ORIENTED_EDGE('',*,*,#7891,.F.);
#10502=ORIENTED_EDGE('',*,*,#7881,.F.);
#10503=ORIENTED_EDGE('',*,*,#7890,.F.);
#10504=ORIENTED_EDGE('',*,*,#7915,.T.);
#10505=ORIENTED_EDGE('',*,*,#7916,.T.);
#10506=ORIENTED_EDGE('',*,*,#7914,.T.);
#10507=ORIENTED_EDGE('',*,*,#7917,.T.);
#10508=ORIENTED_EDGE('',*,*,#7918,.T.);
#10509=ORIENTED_EDGE('',*,*,#7917,.F.);
#10510=ORIENTED_EDGE('',*,*,#7913,.T.);
#10511=ORIENTED_EDGE('',*,*,#7919,.T.);
#10512=ORIENTED_EDGE('',*,*,#7912,.T.);
#10513=ORIENTED_EDGE('',*,*,#7920,.T.);
#10514=ORIENTED_EDGE('',*,*,#7921,.T.);
#10515=ORIENTED_EDGE('',*,*,#7919,.F.);
#10516=ORIENTED_EDGE('',*,*,#7915,.F.);
#10517=ORIENTED_EDGE('',*,*,#7922,.T.);
#10518=ORIENTED_EDGE('',*,*,#7923,.T.);
#10519=ORIENTED_EDGE('',*,*,#7924,.F.);
#10520=ORIENTED_EDGE('',*,*,#7918,.F.);
#10521=ORIENTED_EDGE('',*,*,#7925,.T.);
#10522=ORIENTED_EDGE('',*,*,#7926,.T.);
#10523=ORIENTED_EDGE('',*,*,#7922,.F.);
#10524=ORIENTED_EDGE('',*,*,#7921,.F.);
#10525=ORIENTED_EDGE('',*,*,#7927,.T.);
#10526=ORIENTED_EDGE('',*,*,#7928,.T.);
#10527=ORIENTED_EDGE('',*,*,#7925,.F.);
#10528=ORIENTED_EDGE('',*,*,#7929,.T.);
#10529=ORIENTED_EDGE('',*,*,#7930,.T.);
#10530=ORIENTED_EDGE('',*,*,#7931,.T.);
#10531=ORIENTED_EDGE('',*,*,#7910,.T.);
#10532=ORIENTED_EDGE('',*,*,#7930,.F.);
#10533=ORIENTED_EDGE('',*,*,#7932,.T.);
#10534=ORIENTED_EDGE('',*,*,#7933,.T.);
#10535=ORIENTED_EDGE('',*,*,#7934,.F.);
#10536=ORIENTED_EDGE('',*,*,#7935,.T.);
#10537=ORIENTED_EDGE('',*,*,#7936,.T.);
#10538=ORIENTED_EDGE('',*,*,#7937,.T.);
#10539=ORIENTED_EDGE('',*,*,#7908,.T.);
#10540=ORIENTED_EDGE('',*,*,#7936,.F.);
#10541=ORIENTED_EDGE('',*,*,#7938,.T.);
#10542=ORIENTED_EDGE('',*,*,#7939,.T.);
#10543=ORIENTED_EDGE('',*,*,#7940,.F.);
#10544=ORIENTED_EDGE('',*,*,#7941,.T.);
#10545=ORIENTED_EDGE('',*,*,#7942,.T.);
#10546=ORIENTED_EDGE('',*,*,#7943,.T.);
#10547=ORIENTED_EDGE('',*,*,#7906,.T.);
#10548=ORIENTED_EDGE('',*,*,#7942,.F.);
#10549=ORIENTED_EDGE('',*,*,#7944,.T.);
#10550=ORIENTED_EDGE('',*,*,#7945,.T.);
#10551=ORIENTED_EDGE('',*,*,#7946,.F.);
#10552=ORIENTED_EDGE('',*,*,#7947,.T.);
#10553=ORIENTED_EDGE('',*,*,#7948,.T.);
#10554=ORIENTED_EDGE('',*,*,#7949,.T.);
#10555=ORIENTED_EDGE('',*,*,#7904,.T.);
#10556=ORIENTED_EDGE('',*,*,#7948,.F.);
#10557=ORIENTED_EDGE('',*,*,#7950,.T.);
#10558=ORIENTED_EDGE('',*,*,#7951,.T.);
#10559=ORIENTED_EDGE('',*,*,#7952,.F.);
#10560=ORIENTED_EDGE('',*,*,#7953,.F.);
#10561=ORIENTED_EDGE('',*,*,#7954,.F.);
#10562=ORIENTED_EDGE('',*,*,#7955,.F.);
#10563=ORIENTED_EDGE('',*,*,#7956,.T.);
#10564=ORIENTED_EDGE('',*,*,#7900,.T.);
#10565=ORIENTED_EDGE('',*,*,#7954,.T.);
#10566=ORIENTED_EDGE('',*,*,#7957,.T.);
#10567=ORIENTED_EDGE('',*,*,#7958,.F.);
#10568=ORIENTED_EDGE('',*,*,#7959,.F.);
#10569=ORIENTED_EDGE('',*,*,#7960,.F.);
#10570=ORIENTED_EDGE('',*,*,#7961,.T.);
#10571=ORIENTED_EDGE('',*,*,#7962,.T.);
#10572=ORIENTED_EDGE('',*,*,#7959,.T.);
#10573=ORIENTED_EDGE('',*,*,#7898,.T.);
#10574=ORIENTED_EDGE('',*,*,#7963,.T.);
#10575=ORIENTED_EDGE('',*,*,#7964,.T.);
#10576=ORIENTED_EDGE('',*,*,#7960,.T.);
#10577=ORIENTED_EDGE('',*,*,#7965,.T.);
#10578=ORIENTED_EDGE('',*,*,#7966,.T.);
#10579=ORIENTED_EDGE('',*,*,#7958,.T.);
#10580=ORIENTED_EDGE('',*,*,#7967,.T.);
#10581=ORIENTED_EDGE('',*,*,#7955,.T.);
#10582=ORIENTED_EDGE('',*,*,#7899,.T.);
#10583=ORIENTED_EDGE('',*,*,#7968,.T.);
#10584=ORIENTED_EDGE('',*,*,#7969,.T.);
#10585=ORIENTED_EDGE('',*,*,#7953,.T.);
#10586=ORIENTED_EDGE('',*,*,#7970,.T.);
#10587=ORIENTED_EDGE('',*,*,#7971,.T.);
#10588=ORIENTED_EDGE('',*,*,#7957,.F.);
#10589=ORIENTED_EDGE('',*,*,#7969,.F.);
#10590=ORIENTED_EDGE('',*,*,#7972,.F.);
#10591=ORIENTED_EDGE('',*,*,#7973,.T.);
#10592=ORIENTED_EDGE('',*,*,#7974,.F.);
#10593=ORIENTED_EDGE('',*,*,#7968,.F.);
#10594=ORIENTED_EDGE('',*,*,#7975,.F.);
#10595=ORIENTED_EDGE('',*,*,#7976,.T.);
#10596=ORIENTED_EDGE('',*,*,#7977,.T.);
#10597=ORIENTED_EDGE('',*,*,#7972,.T.);
#10598=ORIENTED_EDGE('',*,*,#7978,.T.);
#10599=ORIENTED_EDGE('',*,*,#7979,.T.);
#10600=ORIENTED_EDGE('',*,*,#7973,.F.);
#10601=ORIENTED_EDGE('',*,*,#7977,.F.);
#10602=ORIENTED_EDGE('',*,*,#7980,.T.);
#10603=ORIENTED_EDGE('',*,*,#7978,.F.);
#10604=ORIENTED_EDGE('',*,*,#7981,.F.);
#10605=ORIENTED_EDGE('',*,*,#7982,.F.);
#10606=ORIENTED_EDGE('',*,*,#7983,.T.);
#10607=ORIENTED_EDGE('',*,*,#7984,.F.);
#10608=ORIENTED_EDGE('',*,*,#7985,.F.);
#10609=ORIENTED_EDGE('',*,*,#7986,.F.);
#10610=ORIENTED_EDGE('',*,*,#7987,.F.);
#10611=ORIENTED_EDGE('',*,*,#7980,.F.);
#10612=ORIENTED_EDGE('',*,*,#7976,.F.);
#10613=ORIENTED_EDGE('',*,*,#7988,.F.);
#10614=ORIENTED_EDGE('',*,*,#7989,.F.);
#10615=ORIENTED_EDGE('',*,*,#7990,.F.);
#10616=ORIENTED_EDGE('',*,*,#7985,.T.);
#10617=ORIENTED_EDGE('',*,*,#7991,.F.);
#10618=ORIENTED_EDGE('',*,*,#7981,.T.);
#10619=ORIENTED_EDGE('',*,*,#7992,.F.);
#10620=ORIENTED_EDGE('',*,*,#7993,.F.);
#10621=ORIENTED_EDGE('',*,*,#7994,.T.);
#10622=ORIENTED_EDGE('',*,*,#7995,.T.);
#10623=ORIENTED_EDGE('',*,*,#7986,.T.);
#10624=ORIENTED_EDGE('',*,*,#7990,.T.);
#10625=ORIENTED_EDGE('',*,*,#7996,.T.);
#10626=ORIENTED_EDGE('',*,*,#7997,.T.);
#10627=ORIENTED_EDGE('',*,*,#7920,.F.);
#10628=ORIENTED_EDGE('',*,*,#7911,.T.);
#10629=ORIENTED_EDGE('',*,*,#7916,.F.);
#10630=ORIENTED_EDGE('',*,*,#7997,.F.);
#10631=ORIENTED_EDGE('',*,*,#7924,.T.);
#10632=ORIENTED_EDGE('',*,*,#7998,.T.);
#10633=ORIENTED_EDGE('',*,*,#7927,.F.);
#10634=ORIENTED_EDGE('',*,*,#7999,.T.);
#10635=ORIENTED_EDGE('',*,*,#7935,.F.);
#10636=ORIENTED_EDGE('',*,*,#7907,.T.);
#10637=ORIENTED_EDGE('',*,*,#7931,.F.);
#10638=ORIENTED_EDGE('',*,*,#7999,.F.);
#10639=ORIENTED_EDGE('',*,*,#7934,.T.);
#10640=ORIENTED_EDGE('',*,*,#8000,.T.);
#10641=ORIENTED_EDGE('',*,*,#7938,.F.);
#10642=ORIENTED_EDGE('',*,*,#8001,.T.);
#10643=ORIENTED_EDGE('',*,*,#7929,.F.);
#10644=ORIENTED_EDGE('',*,*,#7909,.T.);
#10645=ORIENTED_EDGE('',*,*,#7937,.F.);
#10646=ORIENTED_EDGE('',*,*,#8001,.F.);
#10647=ORIENTED_EDGE('',*,*,#7940,.T.);
#10648=ORIENTED_EDGE('',*,*,#8002,.T.);
#10649=ORIENTED_EDGE('',*,*,#7932,.F.);
#10650=ORIENTED_EDGE('',*,*,#8003,.T.);
#10651=ORIENTED_EDGE('',*,*,#7947,.F.);
#10652=ORIENTED_EDGE('',*,*,#7903,.T.);
#10653=ORIENTED_EDGE('',*,*,#7943,.F.);
#10654=ORIENTED_EDGE('',*,*,#8003,.F.);
#10655=ORIENTED_EDGE('',*,*,#7946,.T.);
#10656=ORIENTED_EDGE('',*,*,#8004,.T.);
#10657=ORIENTED_EDGE('',*,*,#7950,.F.);
#10658=ORIENTED_EDGE('',*,*,#8005,.T.);
#10659=ORIENTED_EDGE('',*,*,#7941,.F.);
#10660=ORIENTED_EDGE('',*,*,#7905,.T.);
#10661=ORIENTED_EDGE('',*,*,#7949,.F.);
#10662=ORIENTED_EDGE('',*,*,#8005,.F.);
#10663=ORIENTED_EDGE('',*,*,#7952,.T.);
#10664=ORIENTED_EDGE('',*,*,#8006,.T.);
#10665=ORIENTED_EDGE('',*,*,#7944,.F.);
#10666=ORIENTED_EDGE('',*,*,#7992,.T.);
#10667=ORIENTED_EDGE('',*,*,#8007,.T.);
#10668=ORIENTED_EDGE('',*,*,#8008,.T.);
#10669=ORIENTED_EDGE('',*,*,#8007,.F.);
#10670=ORIENTED_EDGE('',*,*,#8008,.F.);
#10671=ORIENTED_EDGE('',*,*,#8009,.T.);
#10672=ORIENTED_EDGE('',*,*,#8010,.T.);
#10673=ORIENTED_EDGE('',*,*,#8009,.F.);
#10674=ORIENTED_EDGE('',*,*,#7966,.F.);
#10675=ORIENTED_EDGE('',*,*,#8011,.T.);
#10676=ORIENTED_EDGE('',*,*,#7996,.F.);
#10677=ORIENTED_EDGE('',*,*,#7989,.T.);
#10678=ORIENTED_EDGE('',*,*,#8012,.T.);
#10679=ORIENTED_EDGE('',*,*,#7962,.F.);
#10680=ORIENTED_EDGE('',*,*,#8013,.F.);
#10681=ORIENTED_EDGE('',*,*,#7994,.F.);
#10682=ORIENTED_EDGE('',*,*,#8011,.F.);
#10683=ORIENTED_EDGE('',*,*,#7965,.F.);
#10684=ORIENTED_EDGE('',*,*,#7963,.F.);
#10685=ORIENTED_EDGE('',*,*,#8012,.F.);
#10686=ORIENTED_EDGE('',*,*,#7988,.T.);
#10687=ORIENTED_EDGE('',*,*,#7975,.T.);
#10688=ORIENTED_EDGE('',*,*,#7971,.F.);
#10689=ORIENTED_EDGE('',*,*,#8014,.T.);
#10690=ORIENTED_EDGE('',*,*,#7964,.F.);
#10691=ORIENTED_EDGE('',*,*,#8014,.F.);
#10692=ORIENTED_EDGE('',*,*,#7970,.F.);
#10693=ORIENTED_EDGE('',*,*,#7967,.F.);
#10694=ORIENTED_EDGE('',*,*,#7984,.T.);
#10695=ORIENTED_EDGE('',*,*,#8015,.T.);
#10696=ORIENTED_EDGE('',*,*,#7982,.T.);
#10697=ORIENTED_EDGE('',*,*,#7991,.T.);
#10698=ORIENTED_EDGE('',*,*,#8015,.F.);
#10699=ORIENTED_EDGE('',*,*,#7983,.F.);
#10700=ORIENTED_EDGE('',*,*,#8016,.T.);
#10701=ORIENTED_EDGE('',*,*,#8017,.T.);
#10702=ORIENTED_EDGE('',*,*,#8018,.T.);
#10703=ORIENTED_EDGE('',*,*,#8019,.T.);
#10704=ORIENTED_EDGE('',*,*,#8018,.F.);
#10705=ORIENTED_EDGE('',*,*,#8020,.F.);
#10706=ORIENTED_EDGE('',*,*,#8021,.T.);
#10707=ORIENTED_EDGE('',*,*,#8017,.F.);
#10708=ORIENTED_EDGE('',*,*,#8021,.F.);
#10709=ORIENTED_EDGE('',*,*,#8019,.F.);
#10710=ORIENTED_EDGE('',*,*,#8022,.T.);
#10711=ORIENTED_EDGE('',*,*,#7901,.T.);
#10712=ORIENTED_EDGE('',*,*,#7956,.F.);
#10713=ORIENTED_EDGE('',*,*,#7974,.T.);
#10714=ORIENTED_EDGE('',*,*,#7979,.F.);
#10715=ORIENTED_EDGE('',*,*,#7987,.T.);
#10716=ORIENTED_EDGE('',*,*,#7995,.F.);
#10717=ORIENTED_EDGE('',*,*,#8013,.T.);
#10718=ORIENTED_EDGE('',*,*,#7961,.F.);
#10719=ORIENTED_EDGE('',*,*,#7902,.T.);
#10720=ORIENTED_EDGE('',*,*,#8022,.F.);
#10721=ORIENTED_EDGE('',*,*,#7993,.T.);
#10722=ORIENTED_EDGE('',*,*,#8023,.T.);
#10723=ORIENTED_EDGE('',*,*,#8024,.T.);
#10724=ORIENTED_EDGE('',*,*,#8023,.F.);
#10725=ORIENTED_EDGE('',*,*,#8025,.F.);
#10726=ORIENTED_EDGE('',*,*,#8026,.T.);
#10727=ORIENTED_EDGE('',*,*,#8024,.F.);
#10728=ORIENTED_EDGE('',*,*,#8026,.F.);
#10729=ORIENTED_EDGE('',*,*,#8020,.T.);
#10730=ORIENTED_EDGE('',*,*,#8027,.T.);
#10731=ORIENTED_EDGE('',*,*,#8028,.T.);
#10732=ORIENTED_EDGE('',*,*,#8027,.F.);
#10733=ORIENTED_EDGE('',*,*,#8028,.F.);
#10734=ORIENTED_EDGE('',*,*,#8029,.F.);
#10735=ORIENTED_EDGE('',*,*,#8030,.T.);
#10736=ORIENTED_EDGE('',*,*,#8031,.T.);
#10737=ORIENTED_EDGE('',*,*,#8029,.T.);
#10738=ORIENTED_EDGE('',*,*,#8032,.T.);
#10739=ORIENTED_EDGE('',*,*,#8025,.T.);
#10740=ORIENTED_EDGE('',*,*,#8032,.F.);
#10741=ORIENTED_EDGE('',*,*,#8016,.F.);
#10742=ORIENTED_EDGE('',*,*,#8033,.T.);
#10743=ORIENTED_EDGE('',*,*,#8034,.T.);
#10744=ORIENTED_EDGE('',*,*,#8033,.F.);
#10745=ORIENTED_EDGE('',*,*,#8034,.F.);
#10746=ORIENTED_EDGE('',*,*,#8010,.F.);
#10747=ORIENTED_EDGE('',*,*,#8035,.F.);
#10748=ORIENTED_EDGE('',*,*,#8031,.F.);
#10749=ORIENTED_EDGE('',*,*,#8036,.T.);
#10750=ORIENTED_EDGE('',*,*,#8035,.T.);
#10751=ORIENTED_EDGE('',*,*,#8036,.F.);
#10752=ORIENTED_EDGE('',*,*,#8030,.F.);
#10753=ORIENTED_EDGE('',*,*,#8037,.T.);
#10754=ORIENTED_EDGE('',*,*,#8038,.T.);
#10755=ORIENTED_EDGE('',*,*,#8037,.F.);
#10756=ORIENTED_EDGE('',*,*,#8038,.F.);
#10757=ORIENTED_EDGE('',*,*,#7945,.F.);
#10758=ORIENTED_EDGE('',*,*,#8006,.F.);
#10759=ORIENTED_EDGE('',*,*,#7951,.F.);
#10760=ORIENTED_EDGE('',*,*,#8004,.F.);
#10761=ORIENTED_EDGE('',*,*,#7933,.F.);
#10762=ORIENTED_EDGE('',*,*,#8002,.F.);
#10763=ORIENTED_EDGE('',*,*,#7939,.F.);
#10764=ORIENTED_EDGE('',*,*,#8000,.F.);
#10765=ORIENTED_EDGE('',*,*,#7928,.F.);
#10766=ORIENTED_EDGE('',*,*,#7998,.F.);
#10767=ORIENTED_EDGE('',*,*,#7923,.F.);
#10768=ORIENTED_EDGE('',*,*,#7926,.F.);
#10769=ORIENTED_EDGE('',*,*,#7889,.F.);
#10770=ORIENTED_EDGE('',*,*,#8039,.T.);
#10771=ORIENTED_EDGE('',*,*,#8040,.T.);
#10772=ORIENTED_EDGE('',*,*,#7896,.F.);
#10773=ORIENTED_EDGE('',*,*,#7883,.F.);
#10774=ORIENTED_EDGE('',*,*,#7895,.T.);
#10775=ORIENTED_EDGE('',*,*,#8041,.T.);
#10776=ORIENTED_EDGE('',*,*,#8039,.F.);
#10777=ORIENTED_EDGE('',*,*,#7894,.F.);
#10778=ORIENTED_EDGE('',*,*,#7897,.F.);
#10779=ORIENTED_EDGE('',*,*,#8040,.F.);
#10780=ORIENTED_EDGE('',*,*,#8041,.F.);
#15615=PLANE('',#17219);
#15616=PLANE('',#17220);
#15617=PLANE('',#17221);
#15618=PLANE('',#17222);
#15619=PLANE('',#17223);
#15620=PLANE('',#17224);
#15621=PLANE('',#17225);
#15622=PLANE('',#17228);
#15623=PLANE('',#17229);
#15624=PLANE('',#17230);
#15625=PLANE('',#17231);
#15626=PLANE('',#17232);
#15627=PLANE('',#17233);
#15628=PLANE('',#17234);
#15629=PLANE('',#17235);
#15630=PLANE('',#17236);
#15631=PLANE('',#17237);
#15632=PLANE('',#17238);
#15633=PLANE('',#17239);
#15634=PLANE('',#17240);
#15635=PLANE('',#17241);
#15636=PLANE('',#17242);
#15637=PLANE('',#17243);
#15638=PLANE('',#17245);
#15639=PLANE('',#17246);
#15640=PLANE('',#17248);
#15641=PLANE('',#17249);
#15642=PLANE('',#17250);
#15643=PLANE('',#17251);
#15644=PLANE('',#17253);
#15645=PLANE('',#17262);
#15646=PLANE('',#17269);
#15647=PLANE('',#17270);
#15648=PLANE('',#17271);
#15649=PLANE('',#17272);
#15650=PLANE('',#17273);
#15651=PLANE('',#17274);
#15652=PLANE('',#17275);
#15653=PLANE('',#17276);
#15654=PLANE('',#17277);
#15655=PLANE('',#17278);
#15656=PLANE('',#17283);
#15657=PLANE('',#17284);
#15658=PLANE('',#17286);
#15659=PLANE('',#17287);
#15660=PLANE('',#17288);
#15661=PLANE('',#17289);
#15662=PLANE('',#17303);
#15663=PLANE('',#17310);
#15664=PLANE('',#17311);
#15665=PLANE('',#17316);
#15666=PLANE('',#17317);
#15667=PLANE('',#17318);
#15668=PLANE('',#17319);
#15669=PLANE('',#17320);
#15670=PLANE('',#17321);
#15671=PLANE('',#17322);
#16089=ADVANCED_FACE('',(#2280),#15615,.T.);
#16090=ADVANCED_FACE('',(#2281),#15616,.T.);
#16091=ADVANCED_FACE('',(#2282),#15617,.T.);
#16092=ADVANCED_FACE('',(#2283),#15618,.T.);
#16093=ADVANCED_FACE('',(#2284),#15619,.F.);
#16094=ADVANCED_FACE('',(#2285),#15620,.F.);
#16095=ADVANCED_FACE('',(#2286,#1432,#1433,#1434,#1435),#15621,.T.);
#16096=ADVANCED_FACE('',(#2287),#15622,.T.);
#16097=ADVANCED_FACE('',(#2288),#15623,.T.);
#16098=ADVANCED_FACE('',(#2289),#15624,.T.);
#16099=ADVANCED_FACE('',(#2290),#15625,.F.);
#16100=ADVANCED_FACE('',(#2291),#15626,.F.);
#16101=ADVANCED_FACE('',(#2292),#15627,.F.);
#16102=ADVANCED_FACE('',(#2293),#15628,.T.);
#16103=ADVANCED_FACE('',(#2294),#15629,.F.);
#16104=ADVANCED_FACE('',(#2295),#15630,.T.);
#16105=ADVANCED_FACE('',(#2296),#15631,.F.);
#16106=ADVANCED_FACE('',(#2297),#15632,.T.);
#16107=ADVANCED_FACE('',(#2298),#15633,.F.);
#16108=ADVANCED_FACE('',(#2299),#15634,.T.);
#16109=ADVANCED_FACE('',(#2300),#15635,.F.);
#16110=ADVANCED_FACE('',(#2301),#15636,.T.);
#16111=ADVANCED_FACE('',(#2302),#15637,.T.);
#16112=ADVANCED_FACE('',(#2303),#15638,.T.);
#16113=ADVANCED_FACE('',(#2304),#15639,.T.);
#16114=ADVANCED_FACE('',(#2305),#15640,.T.);
#16115=ADVANCED_FACE('',(#2306),#15641,.T.);
#16116=ADVANCED_FACE('',(#2307),#15642,.T.);
#16117=ADVANCED_FACE('',(#2308),#15643,.T.);
#16118=ADVANCED_FACE('',(#2309),#15644,.T.);
#16119=ADVANCED_FACE('',(#2310),#847,.T.);
#16120=ADVANCED_FACE('',(#2311),#139,.F.);
#16121=ADVANCED_FACE('',(#2312,#1436,#1437),#15645,.F.);
#16122=ADVANCED_FACE('',(#2313),#848,.T.);
#16123=ADVANCED_FACE('',(#2314),#15646,.T.);
#16124=ADVANCED_FACE('',(#2315),#15647,.F.);
#16125=ADVANCED_FACE('',(#2316),#15648,.T.);
#16126=ADVANCED_FACE('',(#2317),#15649,.F.);
#16127=ADVANCED_FACE('',(#2318),#15650,.T.);
#16128=ADVANCED_FACE('',(#2319),#15651,.F.);
#16129=ADVANCED_FACE('',(#2320),#15652,.T.);
#16130=ADVANCED_FACE('',(#2321),#15653,.F.);
#16131=ADVANCED_FACE('',(#2322),#15654,.T.);
#16132=ADVANCED_FACE('',(#2323),#15655,.F.);
#16133=ADVANCED_FACE('',(#2324),#849,.F.);
#16134=ADVANCED_FACE('',(#2325),#140,.F.);
#16135=ADVANCED_FACE('',(#2326),#15656,.T.);
#16136=ADVANCED_FACE('',(#2327),#15657,.T.);
#16137=ADVANCED_FACE('',(#2328),#15658,.T.);
#16138=ADVANCED_FACE('',(#2329),#15659,.T.);
#16139=ADVANCED_FACE('',(#2330),#15660,.T.);
#16140=ADVANCED_FACE('',(#2331,#1438),#15661,.T.);
#16141=ADVANCED_FACE('',(#2332),#850,.T.);
#16142=ADVANCED_FACE('',(#2333),#851,.T.);
#16143=ADVANCED_FACE('',(#2334),#141,.T.);
#16144=ADVANCED_FACE('',(#2335),#852,.F.);
#16145=ADVANCED_FACE('',(#2336),#142,.F.);
#16146=ADVANCED_FACE('',(#2337),#853,.T.);
#16147=ADVANCED_FACE('',(#2338,#1439,#1440,#1441),#15662,.T.);
#16148=ADVANCED_FACE('',(#2339),#854,.F.);
#16149=ADVANCED_FACE('',(#2340),#143,.F.);
#16150=ADVANCED_FACE('',(#2341),#15663,.T.);
#16151=ADVANCED_FACE('',(#2342,#1442),#15664,.F.);
#16152=ADVANCED_FACE('',(#2343),#144,.F.);
#16153=ADVANCED_FACE('',(#2344),#145,.F.);
#16154=ADVANCED_FACE('',(#2345),#15665,.T.);
#16155=ADVANCED_FACE('',(#2346),#15666,.F.);
#16156=ADVANCED_FACE('',(#2347),#15667,.F.);
#16157=ADVANCED_FACE('',(#2348),#15668,.F.);
#16158=ADVANCED_FACE('',(#2349),#15669,.F.);
#16159=ADVANCED_FACE('',(#2350),#15670,.F.);
#16160=ADVANCED_FACE('',(#2351),#15671,.F.);
#17072=CLOSED_SHELL('',(#16089,#16090,#16091,#16092,#16093,#16094,#16095,
#16096,#16097,#16098,#16099,#16100,#16101,#16102,#16103,#16104,#16105,#16106,
#16107,#16108,#16109,#16110,#16111,#16112,#16113,#16114,#16115,#16116,#16117,
#16118,#16119,#16120,#16121,#16122,#16123,#16124,#16125,#16126,#16127,#16128,
#16129,#16130,#16131,#16132,#16133,#16134,#16135,#16136,#16137,#16138,#16139,
#16140,#16141,#16142,#16143,#16144,#16145,#16146,#16147,#16148,#16149,#16150,
#16151,#16152,#16153,#16154,#16155,#16156,#16157,#16158,#16159,#16160));
#17218=AXIS2_PLACEMENT_3D('',#23617,#19027,#19028);
#17219=AXIS2_PLACEMENT_3D('',#23618,#19029,#19030);
#17220=AXIS2_PLACEMENT_3D('',#23627,#19035,#19036);
#17221=AXIS2_PLACEMENT_3D('',#23636,#19041,#19042);
#17222=AXIS2_PLACEMENT_3D('',#23639,#19045,#19046);
#17223=AXIS2_PLACEMENT_3D('',#23642,#19049,#19050);
#17224=AXIS2_PLACEMENT_3D('',#23648,#19054,#19055);
#17225=AXIS2_PLACEMENT_3D('',#23652,#19058,#19059);
#17226=AXIS2_PLACEMENT_3D('',#23661,#19063,#19064);
#17227=AXIS2_PLACEMENT_3D('',#23662,#19065,#19066);
#17228=AXIS2_PLACEMENT_3D('',#23687,#19079,#19080);
#17229=AXIS2_PLACEMENT_3D('',#23693,#19084,#19085);
#17230=AXIS2_PLACEMENT_3D('',#23697,#19088,#19089);
#17231=AXIS2_PLACEMENT_3D('',#23701,#19092,#19093);
#17232=AXIS2_PLACEMENT_3D('',#23707,#19097,#19098);
#17233=AXIS2_PLACEMENT_3D('',#23711,#19101,#19102);
#17234=AXIS2_PLACEMENT_3D('',#23715,#19105,#19106);
#17235=AXIS2_PLACEMENT_3D('',#23721,#19110,#19111);
#17236=AXIS2_PLACEMENT_3D('',#23727,#19115,#19116);
#17237=AXIS2_PLACEMENT_3D('',#23733,#19120,#19121);
#17238=AXIS2_PLACEMENT_3D('',#23739,#19125,#19126);
#17239=AXIS2_PLACEMENT_3D('',#23745,#19130,#19131);
#17240=AXIS2_PLACEMENT_3D('',#23751,#19135,#19136);
#17241=AXIS2_PLACEMENT_3D('',#23757,#19140,#19141);
#17242=AXIS2_PLACEMENT_3D('',#23763,#19145,#19146);
#17243=AXIS2_PLACEMENT_3D('',#23769,#19150,#19151);
#17244=AXIS2_PLACEMENT_3D('',#23771,#19152,#19153);
#17245=AXIS2_PLACEMENT_3D('',#23773,#19155,#19156);
#17246=AXIS2_PLACEMENT_3D('',#23779,#19160,#19161);
#17247=AXIS2_PLACEMENT_3D('',#23781,#19162,#19163);
#17248=AXIS2_PLACEMENT_3D('',#23783,#19165,#19166);
#17249=AXIS2_PLACEMENT_3D('',#23791,#19171,#19172);
#17250=AXIS2_PLACEMENT_3D('',#23793,#19174,#19175);
#17251=AXIS2_PLACEMENT_3D('',#23801,#19180,#19181);
#17252=AXIS2_PLACEMENT_3D('',#23808,#19183,#19184);
#17253=AXIS2_PLACEMENT_3D('',#23809,#19185,#19186);
#17254=AXIS2_PLACEMENT_3D('',#23814,#19189,#19190);
#17255=AXIS2_PLACEMENT_3D('',#23815,#19191,#19192);
#17256=AXIS2_PLACEMENT_3D('',#23824,#19193,#19194);
#17257=AXIS2_PLACEMENT_3D('',#23825,#19195,#19196);
#17258=AXIS2_PLACEMENT_3D('',#23826,#19197,#19198);
#17259=AXIS2_PLACEMENT_3D('',#23830,#19200,#19201);
#17260=AXIS2_PLACEMENT_3D('',#23832,#19202,#19203);
#17261=AXIS2_PLACEMENT_3D('',#23834,#19204,#19205);
#17262=AXIS2_PLACEMENT_3D('',#23875,#19207,#19208);
#17263=AXIS2_PLACEMENT_3D('',#23880,#19211,#19212);
#17264=AXIS2_PLACEMENT_3D('',#23883,#19214,#19215);
#17265=AXIS2_PLACEMENT_3D('',#23885,#19216,#19217);
#17266=AXIS2_PLACEMENT_3D('',#23886,#19218,#19219);
#17267=AXIS2_PLACEMENT_3D('',#23892,#19220,#19221);
#17268=AXIS2_PLACEMENT_3D('',#23893,#19222,#19223);
#17269=AXIS2_PLACEMENT_3D('',#23894,#19224,#19225);
#17270=AXIS2_PLACEMENT_3D('',#23896,#19227,#19228);
#17271=AXIS2_PLACEMENT_3D('',#23898,#19230,#19231);
#17272=AXIS2_PLACEMENT_3D('',#23900,#19233,#19234);
#17273=AXIS2_PLACEMENT_3D('',#23902,#19236,#19237);
#17274=AXIS2_PLACEMENT_3D('',#23904,#19239,#19240);
#17275=AXIS2_PLACEMENT_3D('',#23906,#19242,#19243);
#17276=AXIS2_PLACEMENT_3D('',#23908,#19245,#19246);
#17277=AXIS2_PLACEMENT_3D('',#23910,#19248,#19249);
#17278=AXIS2_PLACEMENT_3D('',#23912,#19251,#19252);
#17279=AXIS2_PLACEMENT_3D('',#23914,#19254,#19255);
#17280=AXIS2_PLACEMENT_3D('',#23917,#19257,#19258);
#17281=AXIS2_PLACEMENT_3D('',#23918,#19259,#19260);
#17282=AXIS2_PLACEMENT_3D('',#23921,#19262,#19263);
#17283=AXIS2_PLACEMENT_3D('',#23922,#19264,#19265);
#17284=AXIS2_PLACEMENT_3D('',#23925,#19268,#19269);
#17285=AXIS2_PLACEMENT_3D('',#23926,#19270,#19271);
#17286=AXIS2_PLACEMENT_3D('',#23927,#19272,#19273);
#17287=AXIS2_PLACEMENT_3D('',#23929,#19275,#19276);
#17288=AXIS2_PLACEMENT_3D('',#23930,#19277,#19278);
#17289=AXIS2_PLACEMENT_3D('',#23932,#19280,#19281);
#17290=AXIS2_PLACEMENT_3D('',#23934,#19282,#19283);
#17291=AXIS2_PLACEMENT_3D('',#23935,#19284,#19285);
#17292=AXIS2_PLACEMENT_3D('',#23937,#19286,#19287);
#17293=AXIS2_PLACEMENT_3D('',#23940,#19289,#19290);
#17294=AXIS2_PLACEMENT_3D('',#23941,#19291,#19292);
#17295=AXIS2_PLACEMENT_3D('',#23943,#19293,#19294);
#17296=AXIS2_PLACEMENT_3D('',#23945,#19296,#19297);
#17297=AXIS2_PLACEMENT_3D('',#23947,#19299,#19300);
#17298=AXIS2_PLACEMENT_3D('',#23950,#19302,#19303);
#17299=AXIS2_PLACEMENT_3D('',#23951,#19304,#19305);
#17300=AXIS2_PLACEMENT_3D('',#23953,#19306,#19307);
#17301=AXIS2_PLACEMENT_3D('',#23955,#19309,#19310);
#17302=AXIS2_PLACEMENT_3D('',#23958,#19312,#19313);
#17303=AXIS2_PLACEMENT_3D('',#23959,#19314,#19315);
#17304=AXIS2_PLACEMENT_3D('',#23961,#19316,#19317);
#17305=AXIS2_PLACEMENT_3D('',#23963,#19318,#19319);
#17306=AXIS2_PLACEMENT_3D('',#23965,#19320,#19321);
#17307=AXIS2_PLACEMENT_3D('',#23966,#19322,#19323);
#17308=AXIS2_PLACEMENT_3D('',#23968,#19325,#19326);
#17309=AXIS2_PLACEMENT_3D('',#23971,#19328,#19329);
#17310=AXIS2_PLACEMENT_3D('',#23972,#19330,#19331);
#17311=AXIS2_PLACEMENT_3D('',#23973,#19332,#19333);
#17312=AXIS2_PLACEMENT_3D('',#23975,#19334,#19335);
#17313=AXIS2_PLACEMENT_3D('',#23976,#19336,#19337);
#17314=AXIS2_PLACEMENT_3D('',#23978,#19339,#19340);
#17315=AXIS2_PLACEMENT_3D('',#23981,#19342,#19343);
#17316=AXIS2_PLACEMENT_3D('',#23982,#19344,#19345);
#17317=AXIS2_PLACEMENT_3D('',#23983,#19346,#19347);
#17318=AXIS2_PLACEMENT_3D('',#23984,#19348,#19349);
#17319=AXIS2_PLACEMENT_3D('',#23985,#19350,#19351);
#17320=AXIS2_PLACEMENT_3D('',#23986,#19352,#19353);
#17321=AXIS2_PLACEMENT_3D('',#23990,#19356,#19357);
#17322=AXIS2_PLACEMENT_3D('',#23992,#19359,#19360);
#19027=DIRECTION('axis',(0.,0.,1.));
#19028=DIRECTION('refdir',(1.,0.,0.));
#19029=DIRECTION('center_axis',(0.,-0.707106781186548,0.707106781186548));
#19030=DIRECTION('ref_axis',(1.,0.,0.));
#19031=DIRECTION('',(-1.,0.,0.));
#19032=DIRECTION('',(0.577350269189631,-0.577350269189623,-0.577350269189623));
#19033=DIRECTION('',(1.,0.,0.));
#19034=DIRECTION('',(-0.577350269189631,-0.577350269189623,-0.577350269189623));
#19035=DIRECTION('center_axis',(0.,0.707106781186549,0.707106781186546));
#19036=DIRECTION('ref_axis',(1.,0.,0.));
#19037=DIRECTION('',(1.,0.,0.));
#19038=DIRECTION('',(-0.577350269189632,0.577350269189622,-0.577350269189624));
#19039=DIRECTION('',(-1.,0.,0.));
#19040=DIRECTION('',(-0.577350269189632,-0.577350269189622,0.577350269189624));
#19041=DIRECTION('center_axis',(-0.707106781186543,0.,0.707106781186552));
#19042=DIRECTION('ref_axis',(0.707106781186552,0.,0.707106781186543));
#19043=DIRECTION('',(0.,-1.,0.));
#19044=DIRECTION('',(0.,1.,0.));
#19045=DIRECTION('center_axis',(0.707106781186543,0.,0.707106781186552));
#19046=DIRECTION('ref_axis',(0.707106781186552,0.,-0.707106781186543));
#19047=DIRECTION('',(0.,-1.,0.));
#19048=DIRECTION('',(0.,1.,0.));
#19049=DIRECTION('center_axis',(-1.,0.,0.));
#19050=DIRECTION('ref_axis',(0.,1.,0.));
#19051=DIRECTION('',(0.,0.,-1.));
#19052=DIRECTION('',(0.,1.,0.));
#19053=DIRECTION('',(0.,0.,-1.));
#19054=DIRECTION('center_axis',(0.,-1.,0.));
#19055=DIRECTION('ref_axis',(-1.,0.,0.));
#19056=DIRECTION('',(0.,0.,-1.));
#19057=DIRECTION('',(-1.,0.,0.));
#19058=DIRECTION('center_axis',(0.,0.,1.));
#19059=DIRECTION('ref_axis',(0.,1.,0.));
#19060=DIRECTION('',(1.,0.,0.));
#19061=DIRECTION('',(0.,1.,0.));
#19062=DIRECTION('',(-1.,0.,0.));
#19063=DIRECTION('center_axis',(0.,0.,1.));
#19064=DIRECTION('ref_axis',(1.,0.,0.));
#19065=DIRECTION('center_axis',(0.,0.,1.));
#19066=DIRECTION('ref_axis',(1.,0.,0.));
#19067=DIRECTION('',(-1.,0.,0.));
#19068=DIRECTION('',(0.,1.,0.));
#19069=DIRECTION('',(1.,0.,0.));
#19070=DIRECTION('',(0.,-1.,0.));
#19071=DIRECTION('',(-1.,0.,0.));
#19072=DIRECTION('',(0.,1.,0.));
#19073=DIRECTION('',(1.,0.,0.));
#19074=DIRECTION('',(0.,-1.,0.));
#19075=DIRECTION('',(1.,0.,0.));
#19076=DIRECTION('',(0.,-1.,0.));
#19077=DIRECTION('',(-1.,0.,0.));
#19078=DIRECTION('',(0.,1.,0.));
#19079=DIRECTION('center_axis',(-0.707106781186549,0.,0.707106781186546));
#19080=DIRECTION('ref_axis',(0.707106781186546,0.,0.707106781186549));
#19081=DIRECTION('',(0.,-1.,0.));
#19082=DIRECTION('',(-0.577350269189623,0.577350269189628,-0.577350269189626));
#19083=DIRECTION('',(-0.577350269189625,-0.577350269189625,-0.577350269189627));
#19084=DIRECTION('center_axis',(0.,-0.707106781186549,0.707106781186546));
#19085=DIRECTION('ref_axis',(1.,0.,0.));
#19086=DIRECTION('',(1.,0.,0.));
#19087=DIRECTION('',(0.577350269189618,-0.577350269189629,-0.577350269189631));
#19088=DIRECTION('center_axis',(0.707106781186555,0.,0.70710678118654));
#19089=DIRECTION('ref_axis',(0.70710678118654,0.,-0.707106781186555));
#19090=DIRECTION('',(-0.577350269189616,-0.577350269189632,0.577350269189629));
#19091=DIRECTION('',(0.,1.,0.));
#19092=DIRECTION('center_axis',(1.,0.,0.));
#19093=DIRECTION('ref_axis',(0.,-1.,0.));
#19094=DIRECTION('',(0.,0.,-1.));
#19095=DIRECTION('',(0.,-1.,0.));
#19096=DIRECTION('',(0.,0.,-1.));
#19097=DIRECTION('center_axis',(0.,1.,0.));
#19098=DIRECTION('ref_axis',(1.,0.,0.));
#19099=DIRECTION('',(0.,0.,-1.));
#19100=DIRECTION('',(1.,0.,0.));
#19101=DIRECTION('center_axis',(-1.,0.,0.));
#19102=DIRECTION('ref_axis',(0.,1.,0.));
#19103=DIRECTION('',(0.,0.,-1.));
#19104=DIRECTION('',(0.,1.,0.));
#19105=DIRECTION('center_axis',(0.707106781186555,0.,0.70710678118654));
#19106=DIRECTION('ref_axis',(0.70710678118654,0.,-0.707106781186555));
#19107=DIRECTION('',(-0.577350269189618,-0.577350269189629,0.577350269189631));
#19108=DIRECTION('',(0.,1.,0.));
#19109=DIRECTION('',(0.577350269189617,-0.57735026918963,-0.57735026918963));
#19110=DIRECTION('center_axis',(-1.,0.,0.));
#19111=DIRECTION('ref_axis',(0.,1.,0.));
#19112=DIRECTION('',(0.,0.,-1.));
#19113=DIRECTION('',(0.,1.,0.));
#19114=DIRECTION('',(0.,0.,-1.));
#19115=DIRECTION('center_axis',(-0.707106781186549,0.,0.707106781186546));
#19116=DIRECTION('ref_axis',(0.707106781186546,0.,0.707106781186549));
#19117=DIRECTION('',(0.577350269189624,0.577350269189627,0.577350269189627));
#19118=DIRECTION('',(0.,-1.,0.));
#19119=DIRECTION('',(-0.577350269189625,0.577350269189625,-0.577350269189627));
#19120=DIRECTION('center_axis',(1.,0.,0.));
#19121=DIRECTION('ref_axis',(0.,-1.,0.));
#19122=DIRECTION('',(0.,0.,-1.));
#19123=DIRECTION('',(0.,-1.,0.));
#19124=DIRECTION('',(0.,0.,-1.));
#19125=DIRECTION('center_axis',(0.707106781186543,0.,0.707106781186552));
#19126=DIRECTION('ref_axis',(0.707106781186552,0.,-0.707106781186543));
#19127=DIRECTION('',(-0.57735026918963,-0.577350269189625,0.577350269189622));
#19128=DIRECTION('',(0.,1.,0.));
#19129=DIRECTION('',(0.577350269189632,-0.577350269189622,-0.577350269189624));
#19130=DIRECTION('center_axis',(-1.,0.,0.));
#19131=DIRECTION('ref_axis',(0.,1.,0.));
#19132=DIRECTION('',(0.,0.,-1.));
#19133=DIRECTION('',(0.,1.,0.));
#19134=DIRECTION('',(0.,0.,-1.));
#19135=DIRECTION('center_axis',(-0.707106781186543,0.,0.707106781186552));
#19136=DIRECTION('ref_axis',(0.707106781186552,0.,0.707106781186543));
#19137=DIRECTION('',(0.577350269189632,0.577350269189622,0.577350269189624));
#19138=DIRECTION('',(0.,-1.,0.));
#19139=DIRECTION('',(-0.57735026918963,0.577350269189625,-0.577350269189622));
#19140=DIRECTION('center_axis',(1.,0.,0.));
#19141=DIRECTION('ref_axis',(0.,-1.,0.));
#19142=DIRECTION('',(0.,0.,-1.));
#19143=DIRECTION('',(0.,-1.,0.));
#19144=DIRECTION('',(0.,0.,-1.));
#19145=DIRECTION('center_axis',(-0.750023489558556,-0.572798894755224,0.330705596078447));
#19146=DIRECTION('ref_axis',(0.403449110677542,0.,0.915002084748172));
#19147=DIRECTION('',(-0.627963030199562,0.773682358480754,-0.0841310934092862));
#19148=DIRECTION('',(0.,-0.499999999999999,-0.866025403784439));
#19149=DIRECTION('',(0.627963030199561,-0.459700843380977,0.627963030199552));
#19150=DIRECTION('center_axis',(0.,-0.866025403784439,0.499999999999999));
#19151=DIRECTION('ref_axis',(0.,-0.499999999999999,-0.866025403784439));
#19152=DIRECTION('center_axis',(0.,-0.866025403784439,0.499999999999999));
#19153=DIRECTION('ref_axis',(0.,0.499999999999999,0.866025403784439));
#19154=DIRECTION('',(1.,0.,0.));
#19155=DIRECTION('center_axis',(-0.750023489558558,0.572798894755222,0.330705596078446));
#19156=DIRECTION('ref_axis',(0.40344911067754,0.,0.915002084748173));
#19157=DIRECTION('',(-0.627963030199559,-0.459700843380982,-0.627963030199551));
#19158=DIRECTION('',(0.,-0.499999999999999,0.866025403784439));
#19159=DIRECTION('',(0.627963030199559,0.773682358480756,0.0841310934092859));
#19160=DIRECTION('center_axis',(0.,0.866025403784439,0.499999999999999));
#19161=DIRECTION('ref_axis',(0.,-0.499999999999999,0.866025403784439));
#19162=DIRECTION('center_axis',(0.,0.866025403784439,0.499999999999999));
#19163=DIRECTION('ref_axis',(0.,0.499999999999999,-0.866025403784439));
#19164=DIRECTION('',(-1.,0.,0.));
#19165=DIRECTION('center_axis',(-0.707106781186544,0.612372435695797,-0.353553390593276));
#19166=DIRECTION('ref_axis',(-0.447213595499961,0.,0.894427190999914));
#19167=DIRECTION('',(-0.654653670707978,-0.37796447300922,0.65465367070798));
#19168=DIRECTION('',(0.,0.5,0.866025403784439));
#19169=DIRECTION('',(0.,-0.5,-0.866025403784439));
#19170=DIRECTION('',(-0.447213595499962,-0.774596669241483,-0.447213595499955));
#19171=DIRECTION('center_axis',(-0.707106781186543,0.,0.707106781186552));
#19172=DIRECTION('ref_axis',(0.707106781186552,0.,0.707106781186543));
#19173=DIRECTION('',(0.,-1.,0.));
#19174=DIRECTION('center_axis',(-0.707106781186541,-0.6123724356958,-0.353553390593277));
#19175=DIRECTION('ref_axis',(-0.447213595499965,0.,0.894427190999912));
#19176=DIRECTION('',(0.447213595499965,-0.774596669241481,0.447213595499956));
#19177=DIRECTION('',(0.,-0.5,0.866025403784439));
#19178=DIRECTION('',(0.,0.5,-0.866025403784439));
#19179=DIRECTION('',(0.65465367070798,-0.377964473009213,-0.654653670707982));
#19180=DIRECTION('center_axis',(0.,-0.866025403784439,-0.5));
#19181=DIRECTION('ref_axis',(0.,-0.5,0.866025403784439));
#19182=DIRECTION('',(-1.,0.,0.));
#19183=DIRECTION('center_axis',(0.,-0.866025403784439,-0.5));
#19184=DIRECTION('ref_axis',(0.,0.5,-0.866025403784439));
#19185=DIRECTION('center_axis',(0.,-0.5,-0.866025403784439));
#19186=DIRECTION('ref_axis',(-1.,0.,0.));
#19187=DIRECTION('',(-0.447213595499957,-0.774596669241484,0.447213595499958));
#19188=DIRECTION('',(1.,0.,0.));
#19189=DIRECTION('center_axis',(0.,0.5,0.866025403784439));
#19190=DIRECTION('ref_axis',(-2.8028386894984E-15,0.866025403784439,-0.5));
#19191=DIRECTION('center_axis',(0.,0.,1.));
#19192=DIRECTION('ref_axis',(1.,0.,0.));
#19193=DIRECTION('center_axis',(0.,0.,-1.));
#19194=DIRECTION('ref_axis',(1.,0.,0.));
#19195=DIRECTION('center_axis',(0.,0.,1.));
#19196=DIRECTION('ref_axis',(1.,0.,0.));
#19197=DIRECTION('center_axis',(0.,-1.,0.));
#19198=DIRECTION('ref_axis',(5.0532154980743E-16,0.,1.));
#19199=DIRECTION('',(0.,1.,0.));
#19200=DIRECTION('center_axis',(0.,-0.707106781186549,0.707106781186546));
#19201=DIRECTION('ref_axis',(0.,0.707106781186546,0.707106781186549));
#19202=DIRECTION('center_axis',(0.,-1.,0.));
#19203=DIRECTION('ref_axis',(1.,0.,0.));
#19204=DIRECTION('center_axis',(0.,-0.707106781186549,0.707106781186546));
#19205=DIRECTION('ref_axis',(0.,0.707106781186546,0.707106781186549));
#19206=DIRECTION('',(0.,-1.,0.));
#19207=DIRECTION('center_axis',(0.,0.,1.));
#19208=DIRECTION('ref_axis',(1.,0.,0.));
#19209=DIRECTION('',(0.,-1.,0.));
#19210=DIRECTION('',(-1.,0.,0.));
#19211=DIRECTION('center_axis',(0.,0.,1.));
#19212=DIRECTION('ref_axis',(-1.,0.,0.));
#19213=DIRECTION('',(-1.,0.,0.));
#19214=DIRECTION('center_axis',(0.,0.,-1.));
#19215=DIRECTION('ref_axis',(1.,0.,0.));
#19216=DIRECTION('center_axis',(0.,0.,-1.));
#19217=DIRECTION('ref_axis',(1.,0.,0.));
#19218=DIRECTION('center_axis',(0.,0.,1.));
#19219=DIRECTION('ref_axis',(-1.,0.,0.));
#19220=DIRECTION('center_axis',(0.,0.,-1.));
#19221=DIRECTION('ref_axis',(-1.,0.,0.));
#19222=DIRECTION('center_axis',(0.,-0.499999999999998,0.86602540378444));
#19223=DIRECTION('ref_axis',(3.93732101620015E-15,0.86602540378444,0.499999999999998));
#19224=DIRECTION('center_axis',(0.,0.707106781186546,0.707106781186549));
#19225=DIRECTION('ref_axis',(1.,0.,0.));
#19226=DIRECTION('',(-1.,0.,0.));
#19227=DIRECTION('center_axis',(0.,-1.,0.));
#19228=DIRECTION('ref_axis',(-1.,0.,0.));
#19229=DIRECTION('',(-1.,0.,0.));
#19230=DIRECTION('center_axis',(0.,-0.707106781186548,0.707106781186548));
#19231=DIRECTION('ref_axis',(1.,0.,0.));
#19232=DIRECTION('',(1.,0.,0.));
#19233=DIRECTION('center_axis',(0.,1.,0.));
#19234=DIRECTION('ref_axis',(1.,0.,0.));
#19235=DIRECTION('',(1.,0.,0.));
#19236=DIRECTION('center_axis',(0.,0.707106781186549,0.707106781186546));
#19237=DIRECTION('ref_axis',(1.,0.,0.));
#19238=DIRECTION('',(-1.,0.,0.));
#19239=DIRECTION('center_axis',(0.,-1.,0.));
#19240=DIRECTION('ref_axis',(-1.,0.,0.));
#19241=DIRECTION('',(-1.,0.,0.));
#19242=DIRECTION('center_axis',(0.,-0.707106781186549,0.707106781186546));
#19243=DIRECTION('ref_axis',(1.,0.,0.));
#19244=DIRECTION('',(1.,0.,0.));
#19245=DIRECTION('center_axis',(0.,1.,0.));
#19246=DIRECTION('ref_axis',(1.,0.,0.));
#19247=DIRECTION('',(1.,0.,0.));
#19248=DIRECTION('center_axis',(0.,0.707106781186546,0.707106781186549));
#19249=DIRECTION('ref_axis',(1.,0.,0.));
#19250=DIRECTION('',(-1.,0.,0.));
#19251=DIRECTION('center_axis',(0.,-1.,0.));
#19252=DIRECTION('ref_axis',(-1.,0.,0.));
#19253=DIRECTION('',(-1.,0.,0.));
#19254=DIRECTION('center_axis',(0.,0.,-1.));
#19255=DIRECTION('ref_axis',(1.,0.,0.));
#19256=DIRECTION('',(0.707106781186548,-8.65956056235494E-17,0.707106781186547));
#19257=DIRECTION('center_axis',(0.,0.,1.));
#19258=DIRECTION('ref_axis',(1.,0.,0.));
#19259=DIRECTION('center_axis',(0.,0.,1.));
#19260=DIRECTION('ref_axis',(1.,0.,0.));
#19261=DIRECTION('',(0.,0.,1.));
#19262=DIRECTION('center_axis',(0.,0.,1.));
#19263=DIRECTION('ref_axis',(1.,0.,0.));
#19264=DIRECTION('center_axis',(0.,0.499999999999998,-0.86602540378444));
#19265=DIRECTION('ref_axis',(-1.,0.,0.));
#19266=DIRECTION('',(1.,0.,0.));
#19267=DIRECTION('',(-0.447213595499955,0.774596669241485,0.447213595499957));
#19268=DIRECTION('center_axis',(0.,0.866025403784439,-0.5));
#19269=DIRECTION('ref_axis',(0.,-0.5,-0.866025403784439));
#19270=DIRECTION('center_axis',(0.,0.866025403784439,-0.5));
#19271=DIRECTION('ref_axis',(0.,0.5,0.866025403784439));
#19272=DIRECTION('center_axis',(-0.707106781186549,0.,-0.707106781186546));
#19273=DIRECTION('ref_axis',(-0.707106781186546,0.,0.707106781186549));
#19274=DIRECTION('',(0.,1.,0.));
#19275=DIRECTION('center_axis',(-1.,0.,0.));
#19276=DIRECTION('ref_axis',(0.,0.,1.));
#19277=DIRECTION('center_axis',(0.,0.707106781186549,-0.707106781186546));
#19278=DIRECTION('ref_axis',(-1.,0.,0.));
#19279=DIRECTION('',(1.,0.,0.));
#19280=DIRECTION('center_axis',(0.,1.,0.));
#19281=DIRECTION('ref_axis',(1.,0.,0.));
#19282=DIRECTION('center_axis',(0.,-1.,0.));
#19283=DIRECTION('ref_axis',(1.,0.,0.));
#19284=DIRECTION('center_axis',(0.,3.41806786628767E-15,-1.));
#19285=DIRECTION('ref_axis',(1.,3.05029984904931E-17,0.));
#19286=DIRECTION('center_axis',(0.,0.,-1.));
#19287=DIRECTION('ref_axis',(1.,6.12323399573677E-17,0.));
#19288=DIRECTION('',(-0.382683432365089,3.09934474618468E-15,-0.923879532511287));
#19289=DIRECTION('center_axis',(0.,0.,1.));
#19290=DIRECTION('ref_axis',(1.,0.,0.));
#19291=DIRECTION('center_axis',(0.,0.,-1.));
#19292=DIRECTION('ref_axis',(1.,0.,0.));
#19293=DIRECTION('center_axis',(0.,0.,1.));
#19294=DIRECTION('ref_axis',(1.,6.12323399573677E-17,0.));
#19295=DIRECTION('',(-0.707106781186548,-8.65956056235493E-17,-0.707106781186548));
#19296=DIRECTION('center_axis',(0.,0.,1.));
#19297=DIRECTION('ref_axis',(1.,0.,0.));
#19298=DIRECTION('',(0.,0.,-1.));
#19299=DIRECTION('center_axis',(0.,0.,-1.));
#19300=DIRECTION('ref_axis',(1.,0.,0.));
#19301=DIRECTION('',(0.707106781186546,-8.65956056235491E-17,0.707106781186549));
#19302=DIRECTION('center_axis',(0.,0.,1.));
#19303=DIRECTION('ref_axis',(1.,0.,0.));
#19304=DIRECTION('center_axis',(0.,0.,-1.));
#19305=DIRECTION('ref_axis',(1.,0.,0.));
#19306=DIRECTION('center_axis',(0.,0.,-1.));
#19307=DIRECTION('ref_axis',(1.,0.,0.));
#19308=DIRECTION('',(0.,0.,-1.));
#19309=DIRECTION('center_axis',(0.,-8.23585751082044E-15,-1.));
#19310=DIRECTION('ref_axis',(1.,3.08934278087838E-17,0.));
#19311=DIRECTION('',(0.923879532511287,3.06712541512345E-15,0.38268343236509));
#19312=DIRECTION('center_axis',(0.,0.,-1.));
#19313=DIRECTION('ref_axis',(1.,0.,0.));
#19314=DIRECTION('center_axis',(0.,0.,1.));
#19315=DIRECTION('ref_axis',(1.,0.,0.));
#19316=DIRECTION('center_axis',(0.,0.,1.));
#19317=DIRECTION('ref_axis',(1.,0.,0.));
#19318=DIRECTION('center_axis',(0.,0.,-1.));
#19319=DIRECTION('ref_axis',(1.,0.,0.));
#19320=DIRECTION('center_axis',(0.,0.,-1.));
#19321=DIRECTION('ref_axis',(1.,0.,0.));
#19322=DIRECTION('center_axis',(0.,0.,1.));
#19323=DIRECTION('ref_axis',(1.,0.,0.));
#19324=DIRECTION('',(0.707106781186545,8.6595605623549E-17,-0.70710678118655));
#19325=DIRECTION('center_axis',(0.,-1.,0.));
#19326=DIRECTION('ref_axis',(1.,0.,0.));
#19327=DIRECTION('',(0.,-1.,0.));
#19328=DIRECTION('center_axis',(0.,-1.,0.));
#19329=DIRECTION('ref_axis',(1.,0.,0.));
#19330=DIRECTION('center_axis',(0.,1.,0.));
#19331=DIRECTION('ref_axis',(1.,0.,0.));
#19332=DIRECTION('center_axis',(0.,0.,1.));
#19333=DIRECTION('ref_axis',(1.,0.,0.));
#19334=DIRECTION('center_axis',(0.,0.,-1.));
#19335=DIRECTION('ref_axis',(1.,0.,0.));
#19336=DIRECTION('center_axis',(0.,0.,-1.));
#19337=DIRECTION('ref_axis',(1.,0.,0.));
#19338=DIRECTION('',(0.,0.,-1.));
#19339=DIRECTION('center_axis',(0.,0.,-1.));
#19340=DIRECTION('ref_axis',(1.,0.,0.));
#19341=DIRECTION('',(0.,0.,-1.));
#19342=DIRECTION('center_axis',(0.,0.,-1.));
#19343=DIRECTION('ref_axis',(1.,0.,0.));
#19344=DIRECTION('center_axis',(0.,0.,1.));
#19345=DIRECTION('ref_axis',(1.,0.,0.));
#19346=DIRECTION('center_axis',(0.,0.,-1.));
#19347=DIRECTION('ref_axis',(-1.,0.,0.));
#19348=DIRECTION('center_axis',(0.,0.,-1.));
#19349=DIRECTION('ref_axis',(-1.,0.,0.));
#19350=DIRECTION('center_axis',(0.,0.,-1.));
#19351=DIRECTION('ref_axis',(-1.,0.,0.));
#19352=DIRECTION('center_axis',(1.,0.,0.));
#19353=DIRECTION('ref_axis',(0.,-1.,0.));
#19354=DIRECTION('',(0.,0.,-1.));
#19355=DIRECTION('',(0.,-1.,0.));
#19356=DIRECTION('center_axis',(0.,1.,0.));
#19357=DIRECTION('ref_axis',(1.,0.,0.));
#19358=DIRECTION('',(1.,0.,0.));
#19359=DIRECTION('center_axis',(0.,0.,-1.));
#19360=DIRECTION('ref_axis',(-1.,0.,0.));
#23617=CARTESIAN_POINT('',(0.,0.,0.));
#23618=CARTESIAN_POINT('Origin',(-51.5,17.25,9.75));
#23619=CARTESIAN_POINT('',(-51.5,17.5,10.));
#23620=CARTESIAN_POINT('',(-63.5,17.5,10.));
#23621=CARTESIAN_POINT('',(-51.5,17.5,10.));
#23622=CARTESIAN_POINT('',(-63.,17.,9.5));
#23623=CARTESIAN_POINT('',(-63.5,17.5,10.));
#23624=CARTESIAN_POINT('',(-52.,17.,9.5));
#23625=CARTESIAN_POINT('',(-51.5,17.,9.5));
#23626=CARTESIAN_POINT('',(-51.5,17.5,10.));
#23627=CARTESIAN_POINT('Origin',(-46.,1.75,9.75));
#23628=CARTESIAN_POINT('',(-63.5,1.5,10.));
#23629=CARTESIAN_POINT('',(-51.5,1.5,10.));
#23630=CARTESIAN_POINT('',(-46.,1.5,10.));
#23631=CARTESIAN_POINT('',(-52.,2.,9.5));
#23632=CARTESIAN_POINT('',(-51.5,1.5,10.));
#23633=CARTESIAN_POINT('',(-63.,2.,9.5));
#23634=CARTESIAN_POINT('',(-46.,2.,9.5));
#23635=CARTESIAN_POINT('',(-63.,2.,9.5));
#23636=CARTESIAN_POINT('Origin',(-51.75,-2.5,9.75));
#23637=CARTESIAN_POINT('',(-52.,-2.5,9.5));
#23638=CARTESIAN_POINT('',(-51.5,-2.5,10.));
#23639=CARTESIAN_POINT('Origin',(-63.25,-10.,9.75));
#23640=CARTESIAN_POINT('',(-63.5,-10.,10.));
#23641=CARTESIAN_POINT('',(-63.,-10.,9.5));
#23642=CARTESIAN_POINT('Origin',(-63.,2.,10.));
#23643=CARTESIAN_POINT('',(-63.,2.,4.));
#23644=CARTESIAN_POINT('',(-63.,2.,10.));
#23645=CARTESIAN_POINT('',(-63.,17.,4.));
#23646=CARTESIAN_POINT('',(-63.,17.,4.));
#23647=CARTESIAN_POINT('',(-63.,17.,10.));
#23648=CARTESIAN_POINT('Origin',(-52.,2.,10.));
#23649=CARTESIAN_POINT('',(-52.,2.,4.));
#23650=CARTESIAN_POINT('',(-52.,2.,10.));
#23651=CARTESIAN_POINT('',(-63.,2.,4.));
#23652=CARTESIAN_POINT('Origin',(-40.,-22.,10.));
#23653=CARTESIAN_POINT('',(-79.5,21.5,10.));
#23654=CARTESIAN_POINT('',(-42.9156148738428,21.5,10.));
#23655=CARTESIAN_POINT('',(-40.,21.5,10.));
#23656=CARTESIAN_POINT('',(-79.5,-21.5,10.));
#23657=CARTESIAN_POINT('',(-79.5,-11.,10.));
#23658=CARTESIAN_POINT('',(-42.9156148738428,-21.5,10.));
#23659=CARTESIAN_POINT('',(-40.,-21.5,10.));
#23660=CARTESIAN_POINT('',(-48.,-5.8783046359073E-15,10.));
#23661=CARTESIAN_POINT('Origin',(0.,0.,10.));
#23662=CARTESIAN_POINT('Origin',(0.,0.,10.));
#23663=CARTESIAN_POINT('',(-51.5,-1.5,10.));
#23664=CARTESIAN_POINT('',(-63.5,-1.5,10.));
#23665=CARTESIAN_POINT('',(-51.5,-1.5,10.));
#23666=CARTESIAN_POINT('',(-51.5,-17.5,10.));
#23667=CARTESIAN_POINT('',(-51.5,-12.,10.));
#23668=CARTESIAN_POINT('',(-63.5,-17.5,10.));
#23669=CARTESIAN_POINT('',(-46.,-17.5,10.));
#23670=CARTESIAN_POINT('',(-63.5,-19.5,10.));
#23671=CARTESIAN_POINT('',(-65.5,17.5,10.));
#23672=CARTESIAN_POINT('',(-77.5,17.5,10.));
#23673=CARTESIAN_POINT('',(-58.5,17.5,10.));
#23674=CARTESIAN_POINT('',(-65.5,1.5,10.));
#23675=CARTESIAN_POINT('',(-65.5,-2.5,10.));
#23676=CARTESIAN_POINT('',(-77.5,1.5,10.));
#23677=CARTESIAN_POINT('',(-53.,1.5,10.));
#23678=CARTESIAN_POINT('',(-77.5,-10.,10.));
#23679=CARTESIAN_POINT('',(-77.5,-17.5,10.));
#23680=CARTESIAN_POINT('',(-65.5,-17.5,10.));
#23681=CARTESIAN_POINT('',(-53.,-17.5,10.));
#23682=CARTESIAN_POINT('',(-77.5,-1.5,10.));
#23683=CARTESIAN_POINT('',(-77.5,-19.5,10.));
#23684=CARTESIAN_POINT('',(-65.5,-1.5,10.));
#23685=CARTESIAN_POINT('',(-58.5,-1.5,10.));
#23686=CARTESIAN_POINT('',(-65.5,-12.,10.));
#23687=CARTESIAN_POINT('Origin',(-65.75,-12.,9.75));
#23688=CARTESIAN_POINT('',(-66.,-2.,9.5));
#23689=CARTESIAN_POINT('',(-66.,-17.,9.5));
#23690=CARTESIAN_POINT('',(-66.,-12.,9.5));
#23691=CARTESIAN_POINT('',(-64.5,-18.5,11.));
#23692=CARTESIAN_POINT('',(-65.5,-1.5,10.));
#23693=CARTESIAN_POINT('Origin',(-58.5,-1.75,9.75));
#23694=CARTESIAN_POINT('',(-77.,-2.,9.5));
#23695=CARTESIAN_POINT('',(-58.5,-2.,9.5));
#23696=CARTESIAN_POINT('',(-77.5,-1.5,10.));
#23697=CARTESIAN_POINT('Origin',(-77.25,-19.5,9.75));
#23698=CARTESIAN_POINT('',(-77.,-17.,9.5));
#23699=CARTESIAN_POINT('',(-73.5833333333335,-13.5833333333334,6.08333333333338));
#23700=CARTESIAN_POINT('',(-77.,-19.5,9.5));
#23701=CARTESIAN_POINT('Origin',(-66.,-2.,10.));
#23702=CARTESIAN_POINT('',(-66.,-2.,4.));
#23703=CARTESIAN_POINT('',(-66.,-2.,10.));
#23704=CARTESIAN_POINT('',(-66.,-17.,4.));
#23705=CARTESIAN_POINT('',(-66.,-17.,4.));
#23706=CARTESIAN_POINT('',(-66.,-17.,10.));
#23707=CARTESIAN_POINT('Origin',(-77.,-2.,10.));
#23708=CARTESIAN_POINT('',(-77.,-2.,4.));
#23709=CARTESIAN_POINT('',(-77.,-2.,10.));
#23710=CARTESIAN_POINT('',(-66.,-2.,4.));
#23711=CARTESIAN_POINT('Origin',(-77.,-17.,10.));
#23712=CARTESIAN_POINT('',(-77.,-17.,4.));
#23713=CARTESIAN_POINT('',(-77.,-17.,10.));
#23714=CARTESIAN_POINT('',(-77.,-2.,4.));
#23715=CARTESIAN_POINT('Origin',(-77.25,-10.,9.75));
#23716=CARTESIAN_POINT('',(-77.,2.,9.5));
#23717=CARTESIAN_POINT('',(-75.1666666666668,3.83333333333328,7.66666666666671));
#23718=CARTESIAN_POINT('',(-77.,17.,9.5));
#23719=CARTESIAN_POINT('',(-77.,-10.,9.5));
#23720=CARTESIAN_POINT('',(-69.5833333333335,9.58333333333329,2.08333333333329));
#23721=CARTESIAN_POINT('Origin',(-77.,2.,10.));
#23722=CARTESIAN_POINT('',(-77.,2.,4.));
#23723=CARTESIAN_POINT('',(-77.,2.,10.));
#23724=CARTESIAN_POINT('',(-77.,17.,4.));
#23725=CARTESIAN_POINT('',(-77.,17.,4.));
#23726=CARTESIAN_POINT('',(-77.,17.,10.));
#23727=CARTESIAN_POINT('Origin',(-65.75,-2.5,9.75));
#23728=CARTESIAN_POINT('',(-66.,17.,9.5));
#23729=CARTESIAN_POINT('',(-67.8333333333333,15.1666666666667,7.66666666666666));
#23730=CARTESIAN_POINT('',(-66.,2.,9.5));
#23731=CARTESIAN_POINT('',(-66.,-2.5,9.5));
#23732=CARTESIAN_POINT('',(-62.9166666666667,-1.08333333333333,12.5833333333333));
#23733=CARTESIAN_POINT('Origin',(-66.,17.,10.));
#23734=CARTESIAN_POINT('',(-66.,17.,4.));
#23735=CARTESIAN_POINT('',(-66.,17.,10.));
#23736=CARTESIAN_POINT('',(-66.,2.,4.));
#23737=CARTESIAN_POINT('',(-66.,2.,4.));
#23738=CARTESIAN_POINT('',(-66.,2.,10.));
#23739=CARTESIAN_POINT('Origin',(-63.25,-19.5,9.75));
#23740=CARTESIAN_POINT('',(-63.,-17.,9.5));
#23741=CARTESIAN_POINT('',(-60.75,-14.75,7.24999999999999));
#23742=CARTESIAN_POINT('',(-63.,-2.,9.5));
#23743=CARTESIAN_POINT('',(-63.,-19.5,9.5));
#23744=CARTESIAN_POINT('',(-58.3333333333333,-6.66666666666663,4.83333333333335));
#23745=CARTESIAN_POINT('Origin',(-63.,-17.,10.));
#23746=CARTESIAN_POINT('',(-63.,-17.,4.));
#23747=CARTESIAN_POINT('',(-63.,-17.,10.));
#23748=CARTESIAN_POINT('',(-63.,-2.,4.));
#23749=CARTESIAN_POINT('',(-63.,-2.,4.));
#23750=CARTESIAN_POINT('',(-63.,-2.,10.));
#23751=CARTESIAN_POINT('Origin',(-51.75,-12.,9.75));
#23752=CARTESIAN_POINT('',(-52.,-2.,9.5));
#23753=CARTESIAN_POINT('',(-53.4166666666667,-3.41666666666665,8.08333333333335));
#23754=CARTESIAN_POINT('',(-52.,-17.,9.5));
#23755=CARTESIAN_POINT('',(-52.,-12.,9.5));
#23756=CARTESIAN_POINT('',(-51.6666666666667,-17.3333333333333,9.83333333333334));
#23757=CARTESIAN_POINT('Origin',(-52.,-2.,10.));
#23758=CARTESIAN_POINT('',(-52.,-2.,4.));
#23759=CARTESIAN_POINT('',(-52.,-2.,10.));
#23760=CARTESIAN_POINT('',(-52.,-17.,4.));
#23761=CARTESIAN_POINT('',(-52.,-17.,4.));
#23762=CARTESIAN_POINT('',(-52.,-17.,10.));
#23763=CARTESIAN_POINT('Origin',(-79.5,-21.5,10.));
#23764=CARTESIAN_POINT('',(-79.5,-21.75,9.56698729810778));
#23765=CARTESIAN_POINT('',(-80.,-21.1339745962156,9.5));
#23766=CARTESIAN_POINT('',(-79.5,-21.75,9.56698729810778));
#23767=CARTESIAN_POINT('',(-79.5,-21.5,10.));
#23768=CARTESIAN_POINT('',(-80.,-21.1339745962156,9.5));
#23769=CARTESIAN_POINT('Origin',(-40.,-21.625,9.78349364905389));
#23770=CARTESIAN_POINT('',(-42.7894554767877,-21.75,9.56698729810778));
#23771=CARTESIAN_POINT('Origin',(0.,0.,47.239092362731));
#23772=CARTESIAN_POINT('',(-40.,-21.75,9.56698729810778));
#23773=CARTESIAN_POINT('Origin',(-79.5,21.75,9.56698729810778));
#23774=CARTESIAN_POINT('',(-80.,21.1339745962156,9.5));
#23775=CARTESIAN_POINT('',(-79.5,21.5,10.));
#23776=CARTESIAN_POINT('',(-79.5,21.75,9.56698729810778));
#23777=CARTESIAN_POINT('',(-79.5,21.75,9.56698729810778));
#23778=CARTESIAN_POINT('',(-80.,21.1339745962156,9.5));
#23779=CARTESIAN_POINT('Origin',(-40.,21.625,9.78349364905389));
#23780=CARTESIAN_POINT('',(-42.7894554767877,21.75,9.56698729810778));
#23781=CARTESIAN_POINT('Origin',(0.,0.,47.239092362731));
#23782=CARTESIAN_POINT('',(-40.,21.75,9.56698729810778));
#23783=CARTESIAN_POINT('Origin',(-79.75,17.9509618943233,3.48686027918559));
#23784=CARTESIAN_POINT('',(-79.7165063509461,16.1014973081037,0.216506350946106));
#23785=CARTESIAN_POINT('',(-80.,15.9378221735089,0.5));
#23786=CARTESIAN_POINT('',(-82.202059880349,14.6664623088178,2.70205988034902));
#23787=CARTESIAN_POINT('',(-80.,17.7344555433772,3.61186027918559));
#23788=CARTESIAN_POINT('',(-79.5,16.4764973081037,0.433012701892218));
#23789=CARTESIAN_POINT('',(-79.5,18.1674682452695,3.36186027918558));
#23790=CARTESIAN_POINT('',(-73.1008330249197,27.5601796350596,6.83217967697247));
#23791=CARTESIAN_POINT('Origin',(-79.75,-11.,9.75));
#23792=CARTESIAN_POINT('',(-80.,-11.,9.5));
#23793=CARTESIAN_POINT('Origin',(-79.75,-15.0642105483752,-1.51313972081441));
#23794=CARTESIAN_POINT('',(-79.7165063509461,-16.1014973081037,0.216506350946103));
#23795=CARTESIAN_POINT('',(-79.5,-16.4764973081037,0.433012701892219));
#23796=CARTESIAN_POINT('',(-74.1008330249196,-25.8281288274908,5.83217967697252));
#23797=CARTESIAN_POINT('',(-79.5,-15.2807168993213,-1.63813972081441));
#23798=CARTESIAN_POINT('',(-80.,-15.9378221735089,0.5));
#23799=CARTESIAN_POINT('',(-80.,-14.8477041974291,-1.38813972081441));
#23800=CARTESIAN_POINT('',(-81.4877741660632,-15.078855358239,1.98777416606325));
#23801=CARTESIAN_POINT('Origin',(-40.,-16.2264973081037,1.11022302462516E-15));
#23802=CARTESIAN_POINT('',(-45.0122066014966,-16.4764973081037,0.433012701892212));
#23803=CARTESIAN_POINT('',(-20.,-16.4764973081037,0.433012701892219));
#23804=CARTESIAN_POINT('',(-45.069380727806,-16.5151724426986,0.500000000000003));
#23805=CARTESIAN_POINT('Ctrl Pts',(-45.0122066014946,-16.4764973081024,
0.433012701889958));
#23806=CARTESIAN_POINT('Ctrl Pts',(-45.0407770600794,-16.4958226019871,
0.466485092769431));
#23807=CARTESIAN_POINT('Ctrl Pts',(-45.0693807278045,-16.5151724426975,
0.499999999998238));
#23808=CARTESIAN_POINT('Origin',(0.,0.,-28.1051177665153));
#23809=CARTESIAN_POINT('Origin',(-20.,-16.1014973081037,0.216506350946109));
#23810=CARTESIAN_POINT('',(-79.5,-15.7264973081037,0.));
#23811=CARTESIAN_POINT('',(-70.9626933041054,-0.939448351016254,-8.53730669589464));
#23812=CARTESIAN_POINT('',(-44.8210584705248,-15.7264973081037,0.));
#23813=CARTESIAN_POINT('',(-10.,-15.7264973081037,-5.55111512312578E-16));
#23814=CARTESIAN_POINT('Origin',(8.88178419700125E-15,-33.2729580257087,
10.1304538186344));
#23815=CARTESIAN_POINT('Origin',(0.,0.,0.25));
#23816=CARTESIAN_POINT('',(3.3166247903554,47.3840690527945,0.));
#23817=CARTESIAN_POINT('',(3.9686269671671,47.8356561572586,0.500000000251442));
#23818=CARTESIAN_POINT('Ctrl Pts',(3.3166247903554,47.3840690527945,-2.4459601011273E-15));
#23819=CARTESIAN_POINT('Ctrl Pts',(3.46596392094177,47.4729188691332,0.0990603725345726));
#23820=CARTESIAN_POINT('Ctrl Pts',(3.60680863663856,47.5657711324945,0.202162724737091));
#23821=CARTESIAN_POINT('Ctrl Pts',(3.81688656552239,47.7171537854101,0.369509508930015));
#23822=CARTESIAN_POINT('Ctrl Pts',(3.89366123433624,47.7755348972366,0.433886438519603));
#23823=CARTESIAN_POINT('Ctrl Pts',(3.96862696690834,47.8356561575557,0.50000000027468));
#23824=CARTESIAN_POINT('Origin',(0.,0.,0.5));
#23825=CARTESIAN_POINT('Origin',(0.,0.,0.));
#23826=CARTESIAN_POINT('Origin',(0.,49.5,5.));
#23827=CARTESIAN_POINT('',(3.3166247903554,47.,0.));
#23828=CARTESIAN_POINT('',(3.3166247903554,49.5,0.));
#23829=CARTESIAN_POINT('',(3.96862696659689,47.5,0.5));
#23830=CARTESIAN_POINT('Origin',(0.,52.,5.));
#23831=CARTESIAN_POINT('',(-3.96862696659689,47.5,0.5));
#23832=CARTESIAN_POINT('Origin',(0.,47.5,5.));
#23833=CARTESIAN_POINT('',(-3.3166247903554,47.,0.));
#23834=CARTESIAN_POINT('Origin',(0.,52.,5.));
#23835=CARTESIAN_POINT('',(-3.3166247903554,47.3840690527945,0.));
#23836=CARTESIAN_POINT('',(-3.3166247903554,49.5,0.));
#23837=CARTESIAN_POINT('',(-3.9686269671671,47.8356561572586,0.500000000251442));
#23838=CARTESIAN_POINT('Ctrl Pts',(-3.96862696690834,47.8356561575557,0.500000000274678));
#23839=CARTESIAN_POINT('Ctrl Pts',(-3.89366123433624,47.7755348972366,0.4338864385196));
#23840=CARTESIAN_POINT('Ctrl Pts',(-3.8168865655224,47.7171537854101,0.369509508930017));
#23841=CARTESIAN_POINT('Ctrl Pts',(-3.60680863663856,47.5657711324945,0.202162724737091));
#23842=CARTESIAN_POINT('Ctrl Pts',(-3.46596392094177,47.4729188691332,0.0990603725345772));
#23843=CARTESIAN_POINT('Ctrl Pts',(-3.3166247903554,47.3840690527945,1.28369537222284E-15));
#23844=CARTESIAN_POINT('Ctrl Pts',(3.96862696704285,47.8356561572689,0.500000000393301));
#23845=CARTESIAN_POINT('Ctrl Pts',(4.0635320006758,47.8277824767126,0.583698372797031));
#23846=CARTESIAN_POINT('Ctrl Pts',(4.15494510797109,47.8199140758281,0.669663733732518));
#23847=CARTESIAN_POINT('Ctrl Pts',(4.77491092706035,47.7649010053097,1.28962955282178));
#23848=CARTESIAN_POINT('Ctrl Pts',(5.23654048654341,47.7145022029886,1.96378470873662));
#23849=CARTESIAN_POINT('Ctrl Pts',(5.84910641869338,47.6432894697029,3.44182385251829));
#23850=CARTESIAN_POINT('Ctrl Pts',(6.,47.6235235991626,4.24577588428941));
#23851=CARTESIAN_POINT('Ctrl Pts',(6.,47.6235235991626,5.));
#23852=CARTESIAN_POINT('Ctrl Pts',(6.,47.6235235991626,5.75422411571059));
#23853=CARTESIAN_POINT('Ctrl Pts',(5.84910641869338,47.6432894697029,6.55817614748171));
#23854=CARTESIAN_POINT('Ctrl Pts',(5.23654048654341,47.7145022029886,8.03621529126338));
#23855=CARTESIAN_POINT('Ctrl Pts',(4.77491092706036,47.7649010053097,8.71037044717822));
#23856=CARTESIAN_POINT('Ctrl Pts',(3.71037489380949,47.859363303171,9.77490648042908));
#23857=CARTESIAN_POINT('Ctrl Pts',(3.03621780475891,47.9095897499151,10.2365395235958));
#23858=CARTESIAN_POINT('Ctrl Pts',(1.55817211535174,47.980407545225,10.8491080110314));
#23859=CARTESIAN_POINT('Ctrl Pts',(0.754217814857577,48.,11.));
#23860=CARTESIAN_POINT('Ctrl Pts',(-0.754217814857576,48.,11.));
#23861=CARTESIAN_POINT('Ctrl Pts',(-1.55817211535174,47.980407545225,10.8491080110314));
#23862=CARTESIAN_POINT('Ctrl Pts',(-3.0362178047589,47.9095897499151,10.2365395235958));
#23863=CARTESIAN_POINT('Ctrl Pts',(-3.71037489380949,47.859363303171,9.77490648042908));
#23864=CARTESIAN_POINT('Ctrl Pts',(-4.77491092706036,47.7649010053097,8.71037044717822));
#23865=CARTESIAN_POINT('Ctrl Pts',(-5.23654048654341,47.7145022029886,8.03621529126338));
#23866=CARTESIAN_POINT('Ctrl Pts',(-5.84910641869338,47.6432894697029,6.55817614748171));
#23867=CARTESIAN_POINT('Ctrl Pts',(-6.,47.6235235991626,5.75422411571059));
#23868=CARTESIAN_POINT('Ctrl Pts',(-6.,47.6235235991626,4.24577588428941));
#23869=CARTESIAN_POINT('Ctrl Pts',(-5.84910641869338,47.6432894697029,3.44182385251829));
#23870=CARTESIAN_POINT('Ctrl Pts',(-5.23654048654342,47.7145022029886,1.96378470873662));
#23871=CARTESIAN_POINT('Ctrl Pts',(-4.77491092706036,47.7649010053097,1.28962955282179));
#23872=CARTESIAN_POINT('Ctrl Pts',(-4.15494510795552,47.8199140758295,0.66966373371695));
#23873=CARTESIAN_POINT('Ctrl Pts',(-4.06353200066262,47.8277824767137,0.583698372785401));
#23874=CARTESIAN_POINT('Ctrl Pts',(-3.96862696704285,47.8356561572689,0.500000000393302));
#23875=CARTESIAN_POINT('Origin',(0.,0.,0.));
#23876=CARTESIAN_POINT('',(-79.5,15.7264973081037,0.));
#23877=CARTESIAN_POINT('',(-79.5,0.,0.));
#23878=CARTESIAN_POINT('',(-44.8210584705248,15.7264973081037,0.));
#23879=CARTESIAN_POINT('',(-10.,15.7264973081037,0.));
#23880=CARTESIAN_POINT('Origin',(0.,0.,0.));
#23881=CARTESIAN_POINT('',(0.,47.,0.));
#23882=CARTESIAN_POINT('',(13.130339887499,11.7557050458495,0.));
#23883=CARTESIAN_POINT('Origin',(16.1803398874989,11.7557050458495,0.));
#23884=CARTESIAN_POINT('',(19.5,1.40834381901946E-15,0.));
#23885=CARTESIAN_POINT('Origin',(31.,0.,0.));
#23886=CARTESIAN_POINT('Origin',(0.,0.,0.25));
#23887=CARTESIAN_POINT('',(-45.0122066014966,16.4764973081037,0.43301270189222));
#23888=CARTESIAN_POINT('',(-45.069380727806,16.5151724426986,0.500000000000003));
#23889=CARTESIAN_POINT('Ctrl Pts',(-45.0693807278045,16.5151724426975,0.499999999998241));
#23890=CARTESIAN_POINT('Ctrl Pts',(-45.0407770600795,16.4958226019871,0.466485092769441));
#23891=CARTESIAN_POINT('Ctrl Pts',(-45.0122066014947,16.4764973081024,0.433012701889964));
#23892=CARTESIAN_POINT('Origin',(0.,0.,0.5));
#23893=CARTESIAN_POINT('Origin',(2.66453525910038E-14,33.2729580257085,
10.1304538186342));
#23894=CARTESIAN_POINT('Origin',(-53.,-17.25,9.75));
#23895=CARTESIAN_POINT('',(-53.,-17.,9.5));
#23896=CARTESIAN_POINT('Origin',(-66.,-17.,10.));
#23897=CARTESIAN_POINT('',(-77.,-17.,4.));
#23898=CARTESIAN_POINT('Origin',(-58.5,17.25,9.75));
#23899=CARTESIAN_POINT('',(-58.5,17.,9.5));
#23900=CARTESIAN_POINT('Origin',(-77.,17.,10.));
#23901=CARTESIAN_POINT('',(-66.,17.,4.));
#23902=CARTESIAN_POINT('Origin',(-53.,1.75,9.75));
#23903=CARTESIAN_POINT('',(-53.,2.,9.5));
#23904=CARTESIAN_POINT('Origin',(-66.,2.,10.));
#23905=CARTESIAN_POINT('',(-77.,2.,4.));
#23906=CARTESIAN_POINT('Origin',(-51.5,-1.75,9.75));
#23907=CARTESIAN_POINT('',(-51.5,-2.,9.5));
#23908=CARTESIAN_POINT('Origin',(-63.,-2.,10.));
#23909=CARTESIAN_POINT('',(-52.,-2.,4.));
#23910=CARTESIAN_POINT('Origin',(-46.,-17.25,9.75));
#23911=CARTESIAN_POINT('',(-46.,-17.,9.5));
#23912=CARTESIAN_POINT('Origin',(-52.,-17.,10.));
#23913=CARTESIAN_POINT('',(-63.,-17.,4.));
#23914=CARTESIAN_POINT('Origin',(16.1803398874989,11.7557050458495,0.25));
#23915=CARTESIAN_POINT('',(13.630339887499,11.7557050458495,0.5));
#23916=CARTESIAN_POINT('',(13.380339887499,11.7557050458495,0.25));
#23917=CARTESIAN_POINT('Origin',(16.1803398874989,11.7557050458495,0.5));
#23918=CARTESIAN_POINT('Origin',(16.1803398874989,11.7557050458495,0.));
#23919=CARTESIAN_POINT('',(13.630339887499,11.7557050458495,4.));
#23920=CARTESIAN_POINT('',(13.630339887499,11.7557050458495,0.));
#23921=CARTESIAN_POINT('Origin',(16.1803398874989,11.7557050458495,4.));
#23922=CARTESIAN_POINT('Origin',(-20.,16.1014973081037,0.216506350946109));
#23923=CARTESIAN_POINT('',(-20.,16.4764973081037,0.433012701892218));
#23924=CARTESIAN_POINT('',(-70.9626933041054,0.939448351016247,-8.5373066958946));
#23925=CARTESIAN_POINT('Origin',(-40.,22.,10.));
#23926=CARTESIAN_POINT('Origin',(0.,0.,-28.1051177665153));
#23927=CARTESIAN_POINT('Origin',(-79.75,0.,0.25));
#23928=CARTESIAN_POINT('',(-80.,0.,0.5));
#23929=CARTESIAN_POINT('Origin',(-80.,0.,5.));
#23930=CARTESIAN_POINT('Origin',(0.,47.25,0.25));
#23931=CARTESIAN_POINT('',(0.,47.5,0.5));
#23932=CARTESIAN_POINT('Origin',(0.,47.5,5.));
#23933=CARTESIAN_POINT('',(-2.55,47.5,5.));
#23934=CARTESIAN_POINT('Origin',(0.,47.5,5.));
#23935=CARTESIAN_POINT('Origin',(0.,-1.45875170827388E-15,13.1267766952966));
#23936=CARTESIAN_POINT('',(-47.6464466094067,-9.86076131526265E-31,13.5535533905933));
#23937=CARTESIAN_POINT('Origin',(0.,-2.91750341654776E-15,13.5535533905933));
#23938=CARTESIAN_POINT('',(-48.,-5.8783046359073E-15,12.7));
#23939=CARTESIAN_POINT('',(-47.8232233047034,-8.77415915104917E-15,13.1267766952966));
#23940=CARTESIAN_POINT('Origin',(0.,0.,12.7));
#23941=CARTESIAN_POINT('Origin',(0.,0.,13.6));
#23942=CARTESIAN_POINT('',(-47.5535533905933,-1.16472613895746E-14,13.6464466094067));
#23943=CARTESIAN_POINT('Origin',(0.,-2.91181534739364E-15,13.6464466094067));
#23944=CARTESIAN_POINT('',(-47.6,-5.8293187639414E-15,13.6));
#23945=CARTESIAN_POINT('Origin',(0.,0.,0.));
#23946=CARTESIAN_POINT('',(-48.,-5.8783046359073E-15,0.));
#23947=CARTESIAN_POINT('Origin',(31.,0.,0.25));
#23948=CARTESIAN_POINT('',(20.,-1.34711147906209E-15,0.5));
#23949=CARTESIAN_POINT('',(19.75,1.37772764904077E-15,0.25));
#23950=CARTESIAN_POINT('Origin',(31.,0.,0.5));
#23951=CARTESIAN_POINT('Origin',(31.,0.,14.));
#23952=CARTESIAN_POINT('',(20.,1.34711147906209E-15,13.4));
#23953=CARTESIAN_POINT('Origin',(31.,0.,13.4));
#23954=CARTESIAN_POINT('',(20.,1.34711147906209E-15,14.));
#23955=CARTESIAN_POINT('Origin',(0.,-1.45590767369682E-15,13.8232233047034));
#23956=CARTESIAN_POINT('',(-46.7,5.71910055201814E-15,14.));
#23957=CARTESIAN_POINT('',(-47.1267766952966,2.85955027600907E-15,13.8232233047034));
#23958=CARTESIAN_POINT('Origin',(0.,0.,14.));
#23959=CARTESIAN_POINT('Origin',(0.,0.,14.));
#23960=CARTESIAN_POINT('',(19.4,-1.42059028701093E-15,14.));
#23961=CARTESIAN_POINT('Origin',(31.,0.,14.));
#23962=CARTESIAN_POINT('',(-5.,-6.12323399573677E-16,14.));
#23963=CARTESIAN_POINT('Origin',(0.,0.,14.));
#23964=CARTESIAN_POINT('',(14.1303398874989,11.7557050458495,14.));
#23965=CARTESIAN_POINT('Origin',(16.1803398874989,11.7557050458495,14.));
#23966=CARTESIAN_POINT('Origin',(31.,0.,13.7));
#23967=CARTESIAN_POINT('',(19.7,-1.38385088303651E-15,13.7));
#23968=CARTESIAN_POINT('Origin',(0.,47.5,5.));
#23969=CARTESIAN_POINT('',(-2.55,35.5,5.));
#23970=CARTESIAN_POINT('',(-2.55,47.5,5.));
#23971=CARTESIAN_POINT('Origin',(0.,35.5,5.));
#23972=CARTESIAN_POINT('Origin',(0.,35.5,5.));
#23973=CARTESIAN_POINT('Origin',(16.1803398874989,11.7557050458495,4.));
#23974=CARTESIAN_POINT('',(14.1303398874989,11.7557050458495,4.));
#23975=CARTESIAN_POINT('Origin',(16.1803398874989,11.7557050458495,4.));
#23976=CARTESIAN_POINT('Origin',(16.1803398874989,11.7557050458495,14.));
#23977=CARTESIAN_POINT('',(14.1303398874989,11.7557050458495,14.));
#23978=CARTESIAN_POINT('Origin',(0.,0.,14.));
#23979=CARTESIAN_POINT('',(-5.,-6.12323399573677E-16,2.));
#23980=CARTESIAN_POINT('',(-5.,6.12323399573677E-16,14.));
#23981=CARTESIAN_POINT('Origin',(0.,0.,2.));
#23982=CARTESIAN_POINT('Origin',(0.,0.,2.));
#23983=CARTESIAN_POINT('Origin',(-57.5,-9.5,4.));
#23984=CARTESIAN_POINT('Origin',(-71.5,9.5,4.));
#23985=CARTESIAN_POINT('Origin',(-71.5,-9.5,4.));
#23986=CARTESIAN_POINT('Origin',(-52.,17.,10.));
#23987=CARTESIAN_POINT('',(-52.,17.,4.));
#23988=CARTESIAN_POINT('',(-52.,17.,10.));
#23989=CARTESIAN_POINT('',(-52.,2.,4.));
#23990=CARTESIAN_POINT('Origin',(-63.,17.,10.));
#23991=CARTESIAN_POINT('',(-52.,17.,4.));
#23992=CARTESIAN_POINT('Origin',(-57.5,9.5,4.));
#38502=UNCERTAINTY_MEASURE_WITH_UNIT(LENGTH_MEASURE(0.01),#38529,
'DISTANCE_ACCURACY_VALUE',
'Maximum model space distance between geometric entities at asserted c
onnectivities');
#38514=UNCERTAINTY_MEASURE_WITH_UNIT(LENGTH_MEASURE(0.01),#38529,
'DISTANCE_ACCURACY_VALUE',
'Maximum model space distance between geometric entities at asserted c
onnectivities');
#38516=(
GEOMETRIC_REPRESENTATION_CONTEXT(3)
GLOBAL_UNCERTAINTY_ASSIGNED_CONTEXT((#38502))
GLOBAL_UNIT_ASSIGNED_CONTEXT((#38529,#38531,#38532))
REPRESENTATION_CONTEXT('','3D')
);
#38528=(
GEOMETRIC_REPRESENTATION_CONTEXT(3)
GLOBAL_UNCERTAINTY_ASSIGNED_CONTEXT((#38514))
GLOBAL_UNIT_ASSIGNED_CONTEXT((#38529,#38531,#38532))
REPRESENTATION_CONTEXT('','3D')
);
#38529=(
LENGTH_UNIT()
NAMED_UNIT(*)
SI_UNIT(.MILLI.,.METRE.)
);
#38531=(
NAMED_UNIT(*)
PLANE_ANGLE_UNIT()
SI_UNIT($,.RADIAN.)
);
#38532=(
NAMED_UNIT(*)
SI_UNIT($,.STERADIAN.)
SOLID_ANGLE_UNIT()
);
#38534=SHAPE_DEFINITION_REPRESENTATION(#38547,#38576);
#38547=PRODUCT_DEFINITION_SHAPE('',$,#38590);
#38576=SHAPE_REPRESENTATION('',(#17218),#38516);
#38588=PRODUCT_DEFINITION_CONTEXT('part definition',#38629,'design');
#38590=PRODUCT_DEFINITION('2026-10-20-13-39-03-241',
'01_Turret_Base_with_Dovetail',#38603,#38588);
#38603=PRODUCT_DEFINITION_FORMATION('',$,#38632);
#38629=APPLICATION_CONTEXT(
'Core Data for Automotive Mechanical Design Process');
#38630=PRODUCT_CONTEXT('part definition',#38629,'mechanical');
#38632=PRODUCT('2026-10-20-13-39-03-241','01_Turret_Base_with_Dovetail',
$,(#38630));
#38679=COLOUR_RGB('Dark Blue',0.08,0.2,0.34);
#38680=FILL_AREA_STYLE_COLOUR('',#38679);
#38681=FILL_AREA_STYLE('',(#38680));
#38682=SURFACE_STYLE_FILL_AREA(#38681);
#38683=SURFACE_SIDE_STYLE('',(#38682));
#38684=SURFACE_STYLE_USAGE(.BOTH.,#38683);
#38685=PRESENTATION_STYLE_ASSIGNMENT((#38684));
ENDSEC;
END-ISO-10303-21;
